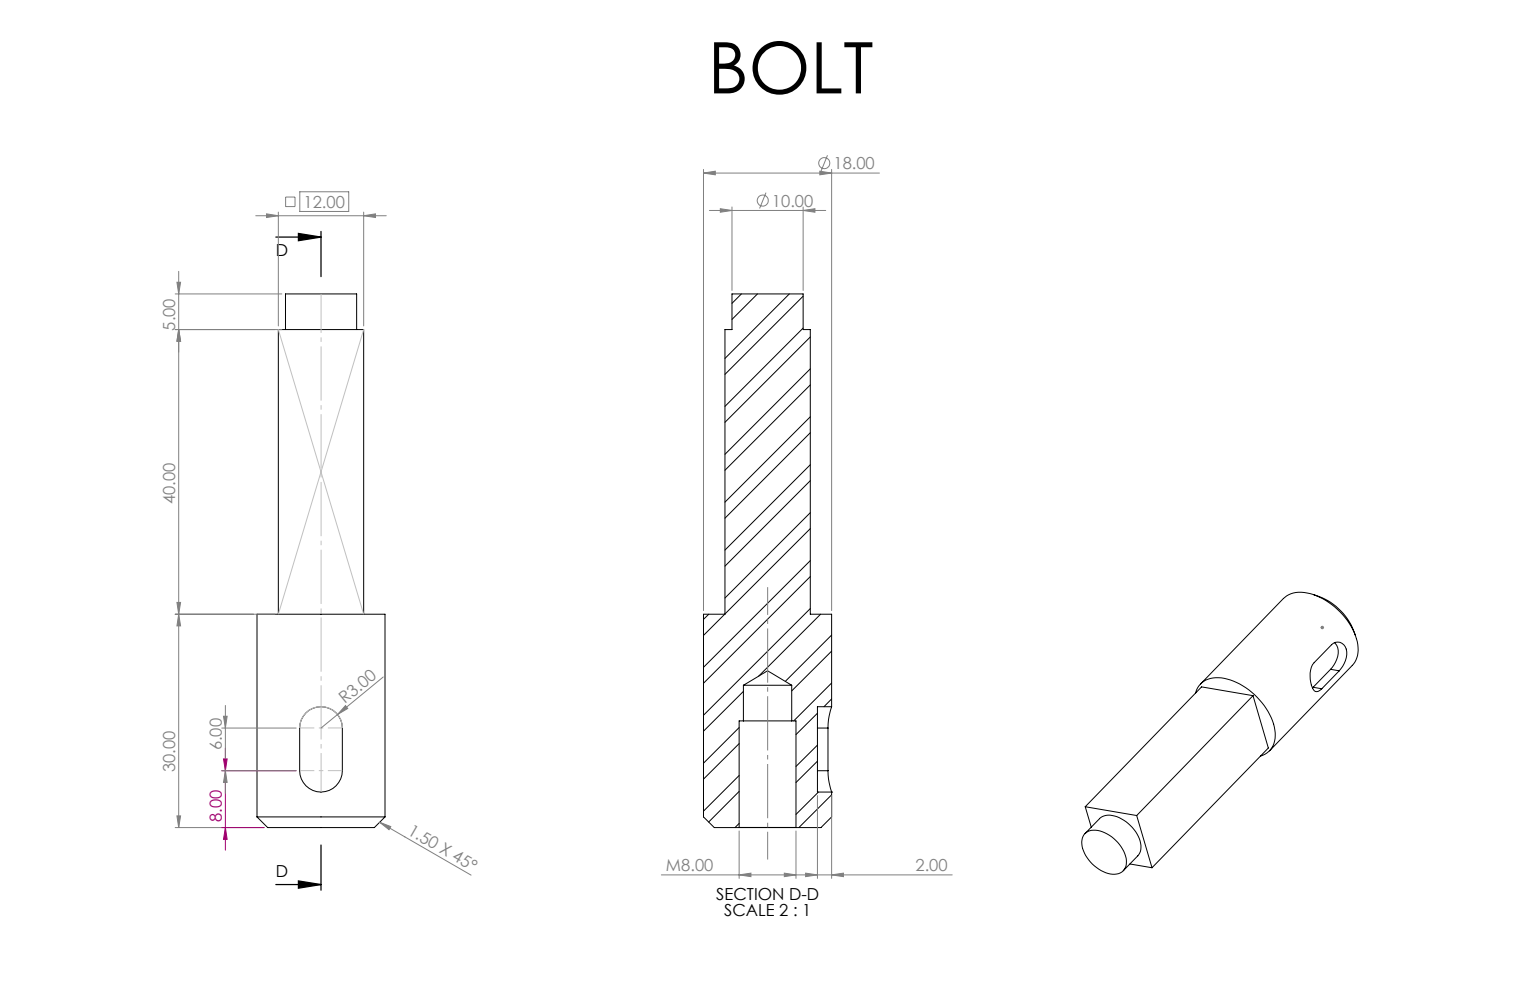
ISO-10303-21;
HEADER;
FILE_DESCRIPTION (('STEP AP214'),
    '1' );
FILE_NAME ('BOLT.step',
    '2026-10-24T00:51:42',
    ( '' ),
    ( '' ),
    'SwSTEP 2.0',
    'SolidWorks 2025',
    '' );
FILE_SCHEMA (( 'AUTOMOTIVE_DESIGN' ));
ENDSEC;

DATA;
#36=CARTESIAN_POINT ( 'NONE',  ( -2.396330562663482766, 23.84645203474120478, 6.679745199209158102 ) ) ;
#83=CIRCLE ( 'NONE', #6686, 8.999999999999998224 ) ;
#86=DIRECTION ( 'NONE',  ( -0.000000000000000000, -1.000000000000000000, -0.000000000000000000 ) ) ;
#93=DIRECTION ( 'NONE',  ( 1.445602896647339163E-16, -0.000000000000000000, 1.000000000000000000 ) ) ;
#98=ORIENTED_EDGE ( 'NONE', *, *, #9067, .T. ) ;
#99=ADVANCED_FACE ( 'NONE', ( #13698 ), #18767, .T. ) ;
#106=CARTESIAN_POINT ( 'NONE',  ( -1.568459684869329074, 24.67391323485165699, 8.880481854261958574 ) ) ;
#156=PLANE ( 'NONE',  #2303 ) ;
#166=FACE_OUTER_BOUND ( 'NONE', #9561, .T. ) ;
#189=EDGE_CURVE ( 'NONE', #17751, #16070, #1466, .T. ) ;
#233=DIRECTION ( 'NONE',  ( 0.000000000000000000, -1.000000000000000000, 0.000000000000000000 ) ) ;
#248=AXIS2_PLACEMENT_3D ( 'NONE', #3692, #16267, #11111 ) ;
#261=CARTESIAN_POINT ( 'NONE',  ( -2.999999999999999112, 30.00000000000000000, 8.485281374238567764 ) ) ;
#308=DIRECTION ( 'NONE',  ( 0.000000000000000000, -1.000000000000000000, 0.000000000000000000 ) ) ;
#314=CARTESIAN_POINT ( 'NONE',  ( -2.999999999999999112, 22.00000000000000355, 8.485281374238567764 ) ) ;
#401=CARTESIAN_POINT ( 'NONE',  ( 5.999999999999999112, -40.00000000000000000, -6.000000000000000000 ) ) ;
#470=ORIENTED_EDGE ( 'NONE', *, *, #21249, .T. ) ;
#514=B_SPLINE_CURVE_WITH_KNOTS ( 'NONE', 3,
 ( #8417, #8302, #13318, #978, #8189, #9907, #4423, #14934, #20459, #1094, #8087, #15044, #13658, #22301, #18383, #11517, #6251, #4767, #6589, #13209, #1429, #17113 ),
 .UNSPECIFIED., .F., .F.,
 ( 4, 2, 2, 2, 2, 2, 2, 2, 2, 2, 4 ),
 ( 0.000000000000000000, 0.1249999999999998612, 0.2499999999999997224, 0.3749999999999995559, 0.4374999999999996114, 0.4999999999999996669, 0.6249999999999996669, 0.7499999999999995559, 0.8749999999999995559, 0.9374999999999998890, 1.000000000000000000 ),
 .UNSPECIFIED. ) ;
#528=VECTOR ( 'NONE', #1528, 1000.000000000000000 ) ;
#533=AXIS2_PLACEMENT_3D ( 'NONE', #17654, #5513, #15925 ) ;
#542=CARTESIAN_POINT ( 'NONE',  ( 1.568459684869332627, 13.32608676514834301, 6.880481854261958574 ) ) ;
#544=DIRECTION ( 'NONE',  ( -0.000000000000000000, 1.000000000000000000, -0.000000000000000000 ) ) ;
#580=VECTOR ( 'NONE', #14375, 1000.000000000000000 ) ;
#666=AXIS2_PLACEMENT_3D ( 'NONE', #5556, #12535, #9120 ) ;
#682=AXIS2_PLACEMENT_3D ( 'NONE', #13089, #4934, #8373 ) ;
#708=ORIENTED_EDGE ( 'NONE', *, *, #21758, .F. ) ;
#722=CARTESIAN_POINT ( 'NONE',  ( -2.673152730111970410, 23.56975547524771741, 8.612623190900162484 ) ) ;
#730=EDGE_CURVE ( 'NONE', #17893, #10226, #5782, .T. ) ;
#783=ORIENTED_EDGE ( 'NONE', *, *, #13913, .T. ) ;
#802=FACE_OUTER_BOUND ( 'NONE', #3383, .T. ) ;
#813=ORIENTED_EDGE ( 'NONE', *, *, #21249, .F. ) ;
#815=EDGE_CURVE ( 'NONE', #15823, #14245, #10221, .T. ) ;
#916=VECTOR ( 'NONE', #20039, 1000.000000000000000 ) ;
#930=EDGE_CURVE ( 'NONE', #7391, #7282, #17354, .T. ) ;
#942=LINE ( 'NONE', #2210, #14631 ) ;
#978=CARTESIAN_POINT ( 'NONE',  ( -2.615521992622583891, 14.48472893833976016, 6.613019222488492943 ) ) ;
#985=CARTESIAN_POINT ( 'NONE',  ( 0.000000000000000000, 9.999999999999998224, 0.000000000000000000 ) ) ;
#1056=CARTESIAN_POINT ( 'NONE',  ( 0.000000000000000000, -40.00000000000000000, 0.000000000000000000 ) ) ;
#1057=CARTESIAN_POINT ( 'NONE',  ( 0.003185071962414435728, 24.99999830921895594, 8.999999436406460163 ) ) ;
#1061=ORIENTED_EDGE ( 'NONE', *, *, #730, .T. ) ;
#1094=CARTESIAN_POINT ( 'NONE',  ( -0.3961047786457937980, 13.02071089460816822, 6.993377406885125325 ) ) ;
#1108=ORIENTED_EDGE ( 'NONE', *, *, #189, .F. ) ;
#1124=DIRECTION ( 'NONE',  ( -0.000000000000000000, 1.000000000000000000, -0.000000000000000000 ) ) ;
#1131=EDGE_LOOP ( 'NONE', ( #16120, #1991 ) ) ;
#1134=ORIENTED_EDGE ( 'NONE', *, *, #7502, .T. ) ;
#1138=EDGE_CURVE ( 'NONE', #16070, #18599, #7758, .T. ) ;
#1211=ORIENTED_EDGE ( 'NONE', *, *, #10301, .T. ) ;
#1231=CARTESIAN_POINT ( 'NONE',  ( 4.929203366568097207E-16, 30.00000000000000355, -4.025000000000000355 ) ) ;
#1292=CARTESIAN_POINT ( 'NONE',  ( 4.898587196589407898E-16, 15.00000000000000355, -3.999999999999994671 ) ) ;
#1324=AXIS2_PLACEMENT_3D ( 'NONE', #6164, #9590, #20145 ) ;
#1347=AXIS2_PLACEMENT_3D ( 'NONE', #14150, #308, #21281 ) ;
#1363=LINE ( 'NONE', #3328, #8712 ) ;
#1385=ORIENTED_EDGE ( 'NONE', *, *, #21758, .T. ) ;
#1393=ORIENTED_EDGE ( 'NONE', *, *, #3282, .F. ) ;
#1429=CARTESIAN_POINT ( 'NONE',  ( 2.999964809120486908, 15.80129619923657103, 6.485293816093339103 ) ) ;
#1466=LINE ( 'NONE', #1231, #11872 ) ;
#1492=VECTOR ( 'NONE', #14249, 1000.000000000000000 ) ;
#1528=DIRECTION ( 'NONE',  ( -1.445602896647339163E-16, -0.000000000000000000, -1.000000000000000000 ) ) ;
#1541=ORIENTED_EDGE ( 'NONE', *, *, #20668, .T. ) ;
#1546=DIRECTION ( 'NONE',  ( 0.000000000000000000, 1.000000000000000000, 0.000000000000000000 ) ) ;
#1556=EDGE_LOOP ( 'NONE', ( #12338, #1541, #14784, #10779 ) ) ;
#1563=VECTOR ( 'NONE', #2236, 1000.000000000000000 ) ;
#1566=B_SPLINE_CURVE_WITH_KNOTS ( 'NONE', 3,
 ( #21891, #18094, #6068, #20054, #2642, #9614 ),
 .UNSPECIFIED., .F., .F.,
 ( 4, 2, 4 ),
 ( 0.5000000000000000000, 0.7500000000000000000, 1.000000000000000000 ),
 .UNSPECIFIED. ) ;
#1580=AXIS2_PLACEMENT_3D ( 'NONE', #3741, #21487, #2586 ) ;
#1593=CONICAL_SURFACE ( 'NONE', #11103, 3.399999999999995026, 1.029744258676652313 ) ;
#1594=EDGE_LOOP ( 'NONE', ( #6227, #6035, #12984, #4629 ) ) ;
#1598=EDGE_CURVE ( 'NONE', #12848, #7247, #8512, .T. ) ;
#1605=CYLINDRICAL_SURFACE ( 'NONE', #682, 3.399999999999995026 ) ;
#1618=EDGE_CURVE ( 'NONE', #18735, #18629, #14479, .T. ) ;
#1648=CARTESIAN_POINT ( 'NONE',  ( 0.000000000000000000, 0.000000000000000000, 0.000000000000000000 ) ) ;
#1653=DIRECTION ( 'NONE',  ( 0.000000000000000000, 1.000000000000000000, 0.000000000000000000 ) ) ;
#1676=ORIENTED_EDGE ( 'NONE', *, *, #17223, .F. ) ;
#1707=EDGE_LOOP ( 'NONE', ( #708, #14419, #2679, #4198, #18260, #21957, #20036, #20335 ) ) ;
#1724=AXIS2_PLACEMENT_3D ( 'NONE', #15557, #93, #5162 ) ;
#1763=( LENGTH_UNIT ( ) NAMED_UNIT ( * ) SI_UNIT ( .MILLI., .METRE. ) );
#1768=CARTESIAN_POINT ( 'NONE',  ( 0.000000000000000000, 30.00000000000000000, 0.000000000000000000 ) ) ;
#1780=ORIENTED_EDGE ( 'NONE', *, *, #6189, .T. ) ;
#1781=CARTESIAN_POINT ( 'NONE',  ( 0.000000000000000000, 30.00000000000000000, 0.000000000000000000 ) ) ;
#1803=EDGE_CURVE ( 'NONE', #13632, #20362, #5094, .T. ) ;
#1843=CARTESIAN_POINT ( 'NONE',  ( 2.999999999999998668, 22.79878727884707956, 6.485281374238567764 ) ) ;
#1865=ORIENTED_EDGE ( 'NONE', *, *, #5944, .F. ) ;
#1891=ADVANCED_FACE ( 'NONE', ( #10334, #3487 ), #6584, .T. ) ;
#1929=FACE_OUTER_BOUND ( 'NONE', #11415, .T. ) ;
#1935=CARTESIAN_POINT ( 'NONE',  ( 0.000000000000000000, -40.00000000000000000, 5.000000000000000000 ) ) ;
#1945=CARTESIAN_POINT ( 'NONE',  ( 2.999999999999998668, 22.79878727884707956, 8.485281374238567764 ) ) ;
#1960=CARTESIAN_POINT ( 'NONE',  ( 0.000000000000000000, 30.00000000000000355, 0.000000000000000000 ) ) ;
#1991=ORIENTED_EDGE ( 'NONE', *, *, #15486, .T. ) ;
#1994=CARTESIAN_POINT ( 'NONE',  ( -2.999999999999998668, 22.00000000000000355, 6.485281374238567764 ) ) ;
#2060=CARTESIAN_POINT ( 'NONE',  ( 0.7921581640248794853, 24.99916066338866116, 6.999720221269573273 ) ) ;
#2073=DIRECTION ( 'NONE',  ( -0.000000000000000000, 1.000000000000000000, -0.000000000000000000 ) ) ;
#2090=ORIENTED_EDGE ( 'NONE', *, *, #14922, .F. ) ;
#2106=AXIS2_PLACEMENT_3D ( 'NONE', #7588, #2317, #7363 ) ;
#2130=DIRECTION ( 'NONE',  ( 0.000000000000000000, 0.000000000000000000, 1.000000000000000000 ) ) ;
#2158=DIRECTION ( 'NONE',  ( -0.000000000000000000, 1.000000000000000000, -0.000000000000000000 ) ) ;
#2171=CARTESIAN_POINT ( 'NONE',  ( 5.999999999999999112, -40.00000000000000000, -6.000000000000000000 ) ) ;
#2210=CARTESIAN_POINT ( 'NONE',  ( -3.000000000000000000, 16.00000000000000000, 8.485281374238567764 ) ) ;
#2236=DIRECTION ( 'NONE',  ( 0.000000000000000000, 0.000000000000000000, -1.000000000000000000 ) ) ;
#2240=ORIENTED_EDGE ( 'NONE', *, *, #12614, .F. ) ;
#2245=PRODUCT_DEFINITION_CONTEXT ( 'detailed design', #5637, 'design' ) ;
#2303=AXIS2_PLACEMENT_3D ( 'NONE', #22413, #10246, #8983 ) ;
#2311=ADVANCED_FACE ( 'NONE', ( #15795 ), #22083, .T. ) ;
#2317=DIRECTION ( 'NONE',  ( 0.000000000000000000, -1.000000000000000000, 0.000000000000000000 ) ) ;
#2331=DIRECTION ( 'NONE',  ( -0.000000000000000000, -1.000000000000000000, -0.000000000000000000 ) ) ;
#2337=ORIENTED_EDGE ( 'NONE', *, *, #18707, .F. ) ;
#2371=EDGE_CURVE ( 'NONE', #4794, #18735, #1566, .T. ) ;
#2417=DIRECTION ( 'NONE',  ( 0.000000000000000000, 0.000000000000000000, 1.000000000000000000 ) ) ;
#2437=ORIENTED_EDGE ( 'NONE', *, *, #11521, .T. ) ;
#2476=DIRECTION ( 'NONE',  ( 0.000000000000000000, 0.7071067811865721087, 0.7071067811865230368 ) ) ;
#2586=DIRECTION ( 'NONE',  ( -1.000000000000000000, 0.000000000000000000, 1.445602896647339163E-16 ) ) ;
#2587=PLANE ( 'NONE',  #8818 ) ;
#2592=ORIENTED_EDGE ( 'NONE', *, *, #16916, .F. ) ;
#2595=CARTESIAN_POINT ( 'NONE',  ( 2.999999999999998668, 22.79878727884707956, 8.485281374238567764 ) ) ;
#2603=ADVANCED_FACE ( 'NONE', ( #17822 ), #21265, .F. ) ;
#2642=CARTESIAN_POINT ( 'NONE',  ( 3.000000000000000444, 15.20112712106396913, 8.485281374238567764 ) ) ;
#2679=ORIENTED_EDGE ( 'NONE', *, *, #3365, .T. ) ;
#2685=ORIENTED_EDGE ( 'NONE', *, *, #6152, .T. ) ;
#2702=CARTESIAN_POINT ( 'NONE',  ( -2.999999999999998668, 22.00000000000000355, 8.485281374238567764 ) ) ;
#2704=CARTESIAN_POINT ( 'NONE',  ( -3.000000000000000000, 16.00000000000000000, 8.485281374238567764 ) ) ;
#2777=DIRECTION ( 'NONE',  ( 0.000000000000000000, -1.000000000000000000, 0.000000000000000000 ) ) ;
#2797=AXIS2_PLACEMENT_3D ( 'NONE', #1781, #5537, #15958 ) ;
#2810=EDGE_LOOP ( 'NONE', ( #18690, #10329 ) ) ;
#2816=CARTESIAN_POINT ( 'NONE',  ( 1.568459684869332627, 13.32608676514834301, 8.880481854261958574 ) ) ;
#2852=EDGE_CURVE ( 'NONE', #11430, #14282, #3269, .T. ) ;
#2860=VECTOR ( 'NONE', #86, 1000.000000000000000 ) ;
#2866=VECTOR ( 'NONE', #10233, 1000.000000000000000 ) ;
#2930=CARTESIAN_POINT ( 'NONE',  ( 2.615521992591937295, 23.51527106174855675, 6.613019222498396132 ) ) ;
#2935=CARTESIAN_POINT ( 'NONE',  ( 3.000000000000000888, 15.99999999999999645, 6.485281374238567764 ) ) ;
#2957=VERTEX_POINT ( 'NONE', #16411 ) ;
#3019=CARTESIAN_POINT ( 'NONE',  ( -6.000000000000000888, 0.000000000000000000, -5.999999999999998224 ) ) ;
#3036=DIRECTION ( 'NONE',  ( 1.000000000000000000, -0.000000000000000000, 0.000000000000000000 ) ) ;
#3045=CARTESIAN_POINT ( 'NONE',  ( -6.000000000000000888, -40.00000000000000000, -5.999999999999998224 ) ) ;
#3073=DIRECTION ( 'NONE',  ( 0.000000000000000000, -0.000000000000000000, -1.000000000000000000 ) ) ;
#3098=VECTOR ( 'NONE', #4298, 1000.000000000000000 ) ;
#3178=DIRECTION ( 'NONE',  ( -0.000000000000000000, 1.000000000000000000, -0.000000000000000000 ) ) ;
#3192=CARTESIAN_POINT ( 'NONE',  ( 0.000000000000000000, -45.00000000000000000, 0.000000000000000000 ) ) ;
#3198=AXIS2_PLACEMENT_3D ( 'NONE', #12267, #10539, #19046 ) ;
#3208=CARTESIAN_POINT ( 'NONE',  ( 0.000000000000000000, 30.00000000000000000, 0.000000000000000000 ) ) ;
#3265=CARTESIAN_POINT ( 'NONE',  ( -1.845281852317813165, 24.39721667535817673, 6.813359845952963845 ) ) ;
#3269=LINE ( 'NONE', #15614, #2866 ) ;
#3282=EDGE_CURVE ( 'NONE', #6865, #17042, #10930, .T. ) ;
#3284=FACE_OUTER_BOUND ( 'NONE', #20720, .T. ) ;
#3328=CARTESIAN_POINT ( 'NONE',  ( 0.000000000000000000, 30.00000000000000000, -7.500000000000000000 ) ) ;
#3347=CYLINDRICAL_SURFACE ( 'NONE', #13196, 8.999999999999998224 ) ;
#3360=DIRECTION ( 'NONE',  ( 1.445602896647339163E-16, 0.000000000000000000, 1.000000000000000000 ) ) ;
#3365=EDGE_CURVE ( 'NONE', #7282, #14700, #4838, .T. ) ;
#3373=ORIENTED_EDGE ( 'NONE', *, *, #9001, .T. ) ;
#3374=CARTESIAN_POINT ( 'NONE',  ( -2.900269772763596876, 22.78549972664023215, 6.519988159899003932 ) ) ;
#3383=EDGE_LOOP ( 'NONE', ( #9239, #2437, #2685, #17262 ) ) ;
#3487=FACE_OUTER_BOUND ( 'NONE', #1131, .T. ) ;
#3592=CIRCLE ( 'NONE', #12346, 5.000000000000000000 ) ;
#3615=VECTOR ( 'NONE', #10576, 1000.000000000000000 ) ;
#3642=EDGE_LOOP ( 'NONE', ( #15490, #98, #17559 ) ) ;
#3683=CARTESIAN_POINT ( 'NONE',  ( -2.673152730111970410, 23.56975547524771741, 6.612623190900161596 ) ) ;
#3692=CARTESIAN_POINT ( 'NONE',  ( 0.000000000000000000, 30.00000000000000000, 0.000000000000000000 ) ) ;
#3699=LINE ( 'NONE', #3045, #10172 ) ;
#3702=ADVANCED_FACE ( 'NONE', ( #802 ), #13255, .F. ) ;
#3705=EDGE_CURVE ( 'NONE', #7282, #7391, #83, .T. ) ;
#3706=ORIENTED_EDGE ( 'NONE', *, *, #4297, .T. ) ;
#3741=CARTESIAN_POINT ( 'NONE',  ( 5.999999999999999112, -40.00000000000000000, -6.000000000000000000 ) ) ;
#3759=EDGE_CURVE ( 'NONE', #3823, #19682, #22455, .T. ) ;
#3761=LINE ( 'NONE', #314, #16607 ) ;
#3821=EDGE_CURVE ( 'NONE', #19682, #15823, #19125, .T. ) ;
#3823=VERTEX_POINT ( 'NONE', #4920 ) ;
#3831=CARTESIAN_POINT ( 'NONE',  ( 0.000000000000000000, 29.97499999999999787, 0.000000000000000000 ) ) ;
#3868=EDGE_CURVE ( 'NONE', #15849, #12848, #19698, .T. ) ;
#3872=CIRCLE ( 'NONE', #17395, 7.500000000000000000 ) ;
#3906=CONICAL_SURFACE ( 'NONE', #1347, 7.500000000000000000, 0.7853981633974447263 ) ;
#4005=PRODUCT_DEFINITION_SHAPE ( 'NONE', 'NONE',  #18657 ) ;
#4023=VERTEX_POINT ( 'NONE', #14625 ) ;
#4028=CARTESIAN_POINT ( 'NONE',  ( -2.673152730111970410, 23.56975547524771741, 8.612623190900162484 ) ) ;
#4081=CARTESIAN_POINT ( 'NONE',  ( 0.000000000000000000, 15.00000000000000000, 0.000000000000000000 ) ) ;
#4177=VECTOR ( 'NONE', #2476, 999.9999999999998863 ) ;
#4198=ORIENTED_EDGE ( 'NONE', *, *, #16916, .T. ) ;
#4285=CARTESIAN_POINT ( 'NONE',  ( 0.000000000000000000, -45.00000000000000000, 5.000000000000000000 ) ) ;
#4297=EDGE_CURVE ( 'NONE', #17042, #6865, #20775, .T. ) ;
#4298=DIRECTION ( 'NONE',  ( 1.049727191138617340E-16, 0.5150380749100560429, -0.8571673007021112234 ) ) ;
#4308=CARTESIAN_POINT ( 'NONE',  ( 4.163799117100996122E-16, 15.00000000000000000, -3.399999999999995914 ) ) ;
#4309=DIRECTION ( 'NONE',  ( 0.000000000000000000, 0.000000000000000000, -1.000000000000000000 ) ) ;
#4399=ORIENTED_EDGE ( 'NONE', *, *, #3759, .T. ) ;
#4423=CARTESIAN_POINT ( 'NONE',  ( -1.516119572518642933, 13.38525031373512064, 6.878942250887981835 ) ) ;
#4425=CARTESIAN_POINT ( 'NONE',  ( 2.673152730111972630, 14.43024452475228614, 6.612623190900158043 ) ) ;
#4434=EDGE_CURVE ( 'NONE', #18399, #11377, #3592, .T. ) ;
#4483=ORIENTED_EDGE ( 'NONE', *, *, #19770, .T. ) ;
#4515=( NAMED_UNIT ( * ) SI_UNIT ( $, .STERADIAN. ) SOLID_ANGLE_UNIT ( ) );
#4538=CARTESIAN_POINT ( 'NONE',  ( -0.7921581640248792633, 13.00083933661134417, 8.999720221269573273 ) ) ;
#4553=EDGE_CURVE ( 'NONE', #17173, #4794, #6860, .T. ) ;
#4586=DIRECTION ( 'NONE',  ( 0.000000000000000000, 0.000000000000000000, 1.000000000000000000 ) ) ;
#4610=ORIENTED_EDGE ( 'NONE', *, *, #7575, .T. ) ;
#4629=ORIENTED_EDGE ( 'NONE', *, *, #930, .F. ) ;
#4647=CARTESIAN_POINT ( 'NONE',  ( 0.000000000000000000, 28.49999999999998934, -8.999999999999998224 ) ) ;
#4724=AXIS2_PLACEMENT_3D ( 'NONE', #6114, #2331, #13076 ) ;
#4731=ORIENTED_EDGE ( 'NONE', *, *, #11521, .F. ) ;
#4748=ORIENTED_EDGE ( 'NONE', *, *, #2371, .T. ) ;
#4767=CARTESIAN_POINT ( 'NONE',  ( 2.842671867368132155, 15.02807304850658987, 6.539645084689668764 ) ) ;
#4793=EDGE_CURVE ( 'NONE', #11430, #19192, #15111, .T. ) ;
#4794=VERTEX_POINT ( 'NONE', #16097 ) ;
#4838=LINE ( 'NONE', #8722, #12759 ) ;
#4872=CARTESIAN_POINT ( 'NONE',  ( -2.670518050928090137, 14.42800760928497539, 8.613211112165400252 ) ) ;
#4889=CARTESIAN_POINT ( 'NONE',  ( -6.000000000000000888, 0.000000000000000000, -5.999999999999998224 ) ) ;
#4907=CARTESIAN_POINT ( 'NONE',  ( 5.999999999999999112, 0.000000000000000000, -6.000000000000000000 ) ) ;
#4920=CARTESIAN_POINT ( 'NONE',  ( -5.999999999999999112, -40.00000000000000000, 6.000000000000001776 ) ) ;
#4934=DIRECTION ( 'NONE',  ( -0.000000000000000000, 1.000000000000000000, -0.000000000000000000 ) ) ;
#4936=EDGE_CURVE ( 'NONE', #20460, #19594, #18693, .T. ) ;
#4942=CARTESIAN_POINT ( 'NONE',  ( -0.003185071962412873176, 13.00000169078104051, 8.999999436406458386 ) ) ;
#4950=VERTEX_POINT ( 'NONE', #2702 ) ;
#4952=CARTESIAN_POINT ( 'NONE',  ( -2.999999999999999112, 16.00000000000000000, 8.485281374238567764 ) ) ;
#4962=EDGE_CURVE ( 'NONE', #4023, #18629, #514, .T. ) ;
#5002=AXIS2_PLACEMENT_3D ( 'NONE', #5712, #9259, #9387 ) ;
#5010=FACE_OUTER_BOUND ( 'NONE', #17802, .T. ) ;
#5046=ORIENTED_EDGE ( 'NONE', *, *, #10998, .T. ) ;
#5067=CARTESIAN_POINT ( 'NONE',  ( -1.572625745558603239, 13.32985487263095159, 8.879522542765043269 ) ) ;
#5094=B_SPLINE_CURVE_WITH_KNOTS ( 'NONE', 3,
 ( #14929, #21954, #6246, #2930, #13202, #9903, #16892, #8185, #15149, #22169, #6469, #13431, #13546, #18840, #3265, #36, #12292, #10564, #3374, #15382, #8410, #5101 ),
 .UNSPECIFIED., .F., .F.,
 ( 4, 2, 2, 2, 2, 2, 2, 2, 2, 2, 4 ),
 ( 0.000000000000000000, 0.1250000000000004163, 0.2500000000000008327, 0.3750000000000012212, 0.4375000000000012212, 0.5000000000000012212, 0.6250000000000012212, 0.7500000000000011102, 0.8750000000000011102, 0.9375000000000005551, 1.000000000000000000 ),
 .UNSPECIFIED. ) ;
#5101=CARTESIAN_POINT ( 'NONE',  ( -2.999999999999998668, 22.00000000000000355, 6.485281374238567764 ) ) ;
#5162=DIRECTION ( 'NONE',  ( 1.000000000000000000, 0.000000000000000000, -1.445602896647339163E-16 ) ) ;
#5349=ORIENTED_EDGE ( 'NONE', *, *, #10128, .T. ) ;
#5451=ORIENTED_EDGE ( 'NONE', *, *, #3821, .F. ) ;
#5461=PLANE ( 'NONE',  #11914 ) ;
#5473=ORIENTED_EDGE ( 'NONE', *, *, #1803, .F. ) ;
#5475=ORIENTED_EDGE ( 'NONE', *, *, #10128, .F. ) ;
#5513=DIRECTION ( 'NONE',  ( -0.000000000000000000, 1.000000000000000000, -0.000000000000000000 ) ) ;
#5537=DIRECTION ( 'NONE',  ( -0.000000000000000000, -1.000000000000000000, -0.000000000000000000 ) ) ;
#5556=CARTESIAN_POINT ( 'NONE',  ( 0.000000000000000000, 30.00000000000000000, 0.000000000000000000 ) ) ;
#5634=ORIENTED_EDGE ( 'NONE', *, *, #3759, .F. ) ;
#5637=APPLICATION_CONTEXT ( 'automotive_design' ) ;
#5694=ORIENTED_EDGE ( 'NONE', *, *, #4553, .T. ) ;
#5696=AXIS2_PLACEMENT_3D ( 'NONE', #9097, #10793, #14580 ) ;
#5708=ORIENTED_EDGE ( 'NONE', *, *, #10301, .F. ) ;
#5712=CARTESIAN_POINT ( 'NONE',  ( 0.000000000000000000, 9.999999999999998224, 0.000000000000000000 ) ) ;
#5728=CARTESIAN_POINT ( 'NONE',  ( 2.999999999999999556, 22.00000000000000000, 6.485281374238567764 ) ) ;
#5767=EDGE_CURVE ( 'NONE', #20460, #7282, #1363, .T. ) ;
#5782=LINE ( 'NONE', #12864, #3098 ) ;
#5821=ADVANCED_FACE ( 'NONE', ( #19126 ), #7241, .T. ) ;
#5854=FACE_OUTER_BOUND ( 'NONE', #10443, .T. ) ;
#5887=FACE_OUTER_BOUND ( 'NONE', #20818, .T. ) ;
#5914=DIRECTION ( 'NONE',  ( -0.000000000000000000, 1.000000000000000000, -0.000000000000000000 ) ) ;
#5937=CARTESIAN_POINT ( 'NONE',  ( 4.929203366568097207E-16, 30.00000000000000355, -4.025000000000000355 ) ) ;
#5944=EDGE_CURVE ( 'NONE', #18599, #16070, #17128, .T. ) ;
#6035=ORIENTED_EDGE ( 'NONE', *, *, #4936, .F. ) ;
#6046=CARTESIAN_POINT ( 'NONE',  ( 5.999999999999999112, -40.00000000000000000, -6.000000000000000000 ) ) ;
#6068=CARTESIAN_POINT ( 'NONE',  ( 1.568459684872858473, 13.32608676515186730, 8.880481854261104147 ) ) ;
#6072=DIRECTION ( 'NONE',  ( 0.000000000000000000, -1.000000000000000000, 0.000000000000000000 ) ) ;
#6094=EDGE_CURVE ( 'NONE', #3823, #18686, #18303, .T. ) ;
#6114=CARTESIAN_POINT ( 'NONE',  ( 0.000000000000000000, 30.00000000000000000, -2.000000000000000000 ) ) ;
#6139=CARTESIAN_POINT ( 'NONE',  ( 2.673152730111972630, 14.43024452475228614, 8.612623190900158932 ) ) ;
#6144=CARTESIAN_POINT ( 'NONE',  ( 0.7921581640149154557, 24.99916066339285692, 8.999720221271109821 ) ) ;
#6152=EDGE_CURVE ( 'NONE', #17751, #14282, #11641, .T. ) ;
#6164=CARTESIAN_POINT ( 'NONE',  ( 0.000000000000000000, 0.000000000000000000, 0.000000000000000000 ) ) ;
#6189=EDGE_CURVE ( 'NONE', #4950, #17173, #13897, .T. ) ;
#6227=ORIENTED_EDGE ( 'NONE', *, *, #10126, .F. ) ;
#6246=CARTESIAN_POINT ( 'NONE',  ( 2.916776610577574314, 22.79308088018310841, 6.515718972866975989 ) ) ;
#6251=CARTESIAN_POINT ( 'NONE',  ( 2.615700731154975145, 14.48345912138648295, 6.612978332551282534 ) ) ;
#6311=ADVANCED_FACE ( 'NONE', ( #5887 ), #21815, .T. ) ;
#6329=DIRECTION ( 'NONE',  ( -0.000000000000000000, 1.000000000000000000, -0.000000000000000000 ) ) ;
#6347=ORIENTED_EDGE ( 'NONE', *, *, #20668, .F. ) ;
#6376=CARTESIAN_POINT ( 'NONE',  ( 6.123233995736766282E-16, -45.00000000000000000, -5.000000000000000000 ) ) ;
#6396=ORIENTED_EDGE ( 'NONE', *, *, #3868, .F. ) ;
#6399=CARTESIAN_POINT ( 'NONE',  ( 0.000000000000000000, 15.00000000000000000, 3.399999999999995470 ) ) ;
#6469=CARTESIAN_POINT ( 'NONE',  ( 0.1993075993174698302, 24.99978691316126955, 6.999930029250658770 ) ) ;
#6502=SHAPE_REPRESENTATION ( 'BOLT', ( #18273 ), #20471 ) ;
#6575=CARTESIAN_POINT ( 'NONE',  ( 6.123233995736766282E-16, -45.00000000000000000, -5.000000000000000000 ) ) ;
#6584=PLANE ( 'NONE',  #7414 ) ;
#6589=CARTESIAN_POINT ( 'NONE',  ( 2.900269772745152519, 15.21450027326556764, 6.519988159905375724 ) ) ;
#6591=CARTESIAN_POINT ( 'NONE',  ( -3.000000000000000000, 16.00000000000000000, 6.485281374238567764 ) ) ;
#6644=EDGE_CURVE ( 'NONE', #4950, #20362, #3761, .T. ) ;
#6685=ORIENTED_EDGE ( 'NONE', *, *, #2371, .F. ) ;
#6686=AXIS2_PLACEMENT_3D ( 'NONE', #21775, #6072, #20059 ) ;
#6703=DIRECTION ( 'NONE',  ( 0.000000000000000000, 1.000000000000000000, 0.000000000000000000 ) ) ;
#6814=ORIENTED_EDGE ( 'NONE', *, *, #7644, .F. ) ;
#6860=B_SPLINE_CURVE_WITH_KNOTS ( 'NONE', 3,
 ( #13515, #18808, #6895, #5067, #10304, #4942 ),
 .UNSPECIFIED., .F., .F.,
 ( 4, 2, 4 ),
 ( 0.000000000000000000, 0.2500000000000000000, 0.5000000000000000000 ),
 .UNSPECIFIED. ) ;
#6865=VERTEX_POINT ( 'NONE', #6376 ) ;
#6874=PLANE ( 'NONE',  #1724 ) ;
#6875=AXIS2_PLACEMENT_3D ( 'NONE', #18101, #14308, #2417 ) ;
#6895=CARTESIAN_POINT ( 'NONE',  ( -2.670518050928090137, 14.42800760928497539, 8.613211112165400252 ) ) ;
#6899=ORIENTED_EDGE ( 'NONE', *, *, #4434, .F. ) ;
#6975=VERTEX_POINT ( 'NONE', #4889 ) ;
#7002=DIRECTION ( 'NONE',  ( -0.000000000000000000, -1.000000000000000000, -0.000000000000000000 ) ) ;
#7035=ORIENTED_EDGE ( 'NONE', *, *, #1803, .T. ) ;
#7067=EDGE_LOOP ( 'NONE', ( #5451, #5634, #17662, #470 ) ) ;
#7082=DIRECTION ( 'NONE',  ( 0.000000000000000000, -1.000000000000000000, 0.000000000000000000 ) ) ;
#7096=LINE ( 'NONE', #7204, #17040 ) ;
#7153=ADVANCED_FACE ( 'NONE', ( #166 ), #12425, .T. ) ;
#7164=ADVANCED_BREP_SHAPE_REPRESENTATION ( '', ( #10851, #18273 ), #20471 ) ;
#7184=EDGE_LOOP ( 'NONE', ( #3706, #17509 ) ) ;
#7188=DIRECTION ( 'NONE',  ( 0.000000000000000000, 0.000000000000000000, -1.000000000000000000 ) ) ;
#7204=CARTESIAN_POINT ( 'NONE',  ( 0.000000000000000000, -45.00000000000000000, 5.000000000000000000 ) ) ;
#7225=ORIENTED_EDGE ( 'NONE', *, *, #1138, .T. ) ;
#7232=VERTEX_POINT ( 'NONE', #401 ) ;
#7241=CONICAL_SURFACE ( 'NONE', #20056, 7.500000000000000000, 0.7853981633974447263 ) ;
#7247=VERTEX_POINT ( 'NONE', #4308 ) ;
#7263=FACE_OUTER_BOUND ( 'NONE', #15492, .T. ) ;
#7282=VERTEX_POINT ( 'NONE', #4647 ) ;
#7286=LINE ( 'NONE', #7624, #1492 ) ;
#7363=DIRECTION ( 'NONE',  ( 0.000000000000000000, 0.000000000000000000, -1.000000000000000000 ) ) ;
#7391=VERTEX_POINT ( 'NONE', #20789 ) ;
#7414=AXIS2_PLACEMENT_3D ( 'NONE', #1768, #20560, #15609 ) ;
#7433=DIRECTION ( 'NONE',  ( 0.000000000000000000, 1.000000000000000000, 0.000000000000000000 ) ) ;
#7451=CARTESIAN_POINT ( 'NONE',  ( -6.000000000000000888, -40.00000000000000000, -5.999999999999998224 ) ) ;
#7502=EDGE_CURVE ( 'NONE', #14282, #17751, #16222, .T. ) ;
#7512=ORIENTED_EDGE ( 'NONE', *, *, #1138, .F. ) ;
#7539=DIRECTION ( 'NONE',  ( 0.000000000000000000, 0.000000000000000000, 1.000000000000000000 ) ) ;
#7567=CYLINDRICAL_SURFACE ( 'NONE', #11988, 5.000000000000000000 ) ;
#7575=EDGE_CURVE ( 'NONE', #14282, #18599, #10942, .T. ) ;
#7579=ADVANCED_FACE ( 'NONE', ( #19439 ), #1593, .F. ) ;
#7588=CARTESIAN_POINT ( 'NONE',  ( 0.000000000000000000, -45.00000000000000000, 0.000000000000000000 ) ) ;
#7595=ORIENTED_EDGE ( 'NONE', *, *, #17800, .F. ) ;
#7624=CARTESIAN_POINT ( 'NONE',  ( 5.999999999999999112, -40.00000000000000000, -6.000000000000000000 ) ) ;
#7644=EDGE_CURVE ( 'NONE', #7232, #17346, #7286, .T. ) ;
#7696=ADVANCED_FACE ( 'NONE', ( #20456 ), #2587, .F. ) ;
#7711=PLANE ( 'NONE',  #19671 ) ;
#7758=CIRCLE ( 'NONE', #16153, 4.025000000000000355 ) ;
#7767=CARTESIAN_POINT ( 'NONE',  ( 4.898587196589408884E-16, 30.00000000000000000, -3.999999999999996447 ) ) ;
#7808=ADVANCED_FACE ( 'NONE', ( #17224, #20904 ), #13774, .F. ) ;
#7835=VECTOR ( 'NONE', #14740, 1000.000000000000000 ) ;
#7846=CARTESIAN_POINT ( 'NONE',  ( 2.999999999999997780, 30.00000000000000000, 8.485281374238567764 ) ) ;
#7851=STYLED_ITEM('',(#22741),#10851);
#7935=DIRECTION ( 'NONE',  ( 0.000000000000000000, 0.000000000000000000, -1.000000000000000000 ) ) ;
#7957=EDGE_CURVE ( 'NONE', #22536, #4950, #18199, .T. ) ;
#8052=EDGE_LOOP ( 'NONE', ( #1676, #17404, #13963, #22249 ) ) ;
#8056=DIRECTION ( 'NONE',  ( 0.000000000000000000, 0.5150380749100560429, 0.8571673007021112234 ) ) ;
#8087=CARTESIAN_POINT ( 'NONE',  ( -0.1993075991723092522, 13.00021308684595311, 6.999930029250709396 ) ) ;
#8094=ADVANCED_FACE ( 'NONE', ( #22482 ), #3347, .T. ) ;
#8116=ORIENTED_EDGE ( 'NONE', *, *, #18280, .F. ) ;
#8118=DIRECTION ( 'NONE',  ( 0.000000000000000000, 0.000000000000000000, 1.000000000000000000 ) ) ;
#8150=ORIENTED_EDGE ( 'NONE', *, *, #15486, .F. ) ;
#8185=CARTESIAN_POINT ( 'NONE',  ( 0.9710767271268372358, 24.84180973946540405, 6.949333411110966807 ) ) ;
#8189=CARTESIAN_POINT ( 'NONE',  ( -2.394928258197305482, 14.15236082731613010, 6.680059847329907541 ) ) ;
#8291=VECTOR ( 'NONE', #9392, 1000.000000000000000 ) ;
#8302=CARTESIAN_POINT ( 'NONE',  ( -2.999929132934958886, 15.60292843345686187, 6.485306429529695826 ) ) ;
#8373=DIRECTION ( 'NONE',  ( 0.000000000000000000, 0.000000000000000000, 1.000000000000000000 ) ) ;
#8410=CARTESIAN_POINT ( 'NONE',  ( -2.999964809119741727, 22.19870380085767891, 6.485293816093604669 ) ) ;
#8417=CARTESIAN_POINT ( 'NONE',  ( -2.999999999999999112, 16.00000000000000000, 6.485281374238567764 ) ) ;
#8453=DIRECTION ( 'NONE',  ( 8.659560562354634570E-17, 0.7071067811865721087, -0.7071067811865230368 ) ) ;
#8478=DIRECTION ( 'NONE',  ( -0.000000000000000000, -1.000000000000000000, -0.000000000000000000 ) ) ;
#8506=CARTESIAN_POINT ( 'NONE',  ( -6.000000000000000888, -40.00000000000000000, -5.999999999999998224 ) ) ;
#8512=CIRCLE ( 'NONE', #17648, 3.399999999999995470 ) ;
#8555=CARTESIAN_POINT ( 'NONE',  ( 4.898587196589410857E-16, 29.97499999999999787, -3.999999999999998224 ) ) ;
#8681=ORIENTED_EDGE ( 'NONE', *, *, #12671, .F. ) ;
#8712=VECTOR ( 'NONE', #17275, 1000.000000000000114 ) ;
#8722=CARTESIAN_POINT ( 'NONE',  ( 0.000000000000000000, 30.00000000000000000, -8.999999999999998224 ) ) ;
#8779=ADVANCED_FACE ( 'NONE', ( #15157 ), #15677, .T. ) ;
#8818=AXIS2_PLACEMENT_3D ( 'NONE', #7846, #3036, #4309 ) ;
#8829=DIRECTION ( 'NONE',  ( 0.000000000000000000, 0.000000000000000000, -1.000000000000000000 ) ) ;
#8906=ADVANCED_FACE ( 'NONE', ( #14453 ), #7711, .T. ) ;
#8912=PLANE ( 'NONE',  #14155 ) ;
#8933=CARTESIAN_POINT ( 'NONE',  ( -0.7857880201000499998, 25.00083595504925071, 9.000278651543347053 ) ) ;
#8940=DIRECTION ( 'NONE',  ( -0.000000000000000000, 1.000000000000000000, -0.000000000000000000 ) ) ;
#8976=CYLINDRICAL_SURFACE ( 'NONE', #2797, 8.999999999999998224 ) ;
#8983=DIRECTION ( 'NONE',  ( 0.000000000000000000, -0.000000000000000000, -1.000000000000000000 ) ) ;
#8990=CONICAL_SURFACE ( 'NONE', #21084, 3.399999999999995026, 1.029744258676652313 ) ;
#9001=EDGE_CURVE ( 'NONE', #20362, #4023, #19863, .T. ) ;
#9003=DIRECTION ( 'NONE',  ( 0.000000000000000000, -1.000000000000000000, 0.000000000000000000 ) ) ;
#9025=CARTESIAN_POINT ( 'NONE',  ( 0.000000000000000000, 9.999999999999998224, 0.000000000000000000 ) ) ;
#9067=EDGE_CURVE ( 'NONE', #17893, #15849, #18253, .T. ) ;
#9093=DIRECTION ( 'NONE',  ( 0.000000000000000000, 0.000000000000000000, -1.000000000000000000 ) ) ;
#9097=CARTESIAN_POINT ( 'NONE',  ( 0.000000000000000000, 30.00000000000000355, 0.000000000000000000 ) ) ;
#9120=DIRECTION ( 'NONE',  ( 0.000000000000000000, 0.000000000000000000, 1.000000000000000000 ) ) ;
#9143=EDGE_CURVE ( 'NONE', #19192, #11430, #10499, .T. ) ;
#9146=DIRECTION ( 'NONE',  ( -1.445602896647339163E-16, 0.000000000000000000, -1.000000000000000000 ) ) ;
#9162=CARTESIAN_POINT ( 'NONE',  ( -2.999999999999999556, 22.00000000000000355, 6.485281374238567764 ) ) ;
#9205=CARTESIAN_POINT ( 'NONE',  ( 0.000000000000000000, 30.00000000000000000, -7.500000000000000000 ) ) ;
#9239=ORIENTED_EDGE ( 'NONE', *, *, #9143, .F. ) ;
#9246=CARTESIAN_POINT ( 'NONE',  ( 3.000000000000000444, 15.20112712106396913, 6.485281374238567764 ) ) ;
#9247=DIRECTION ( 'NONE',  ( 0.000000000000000000, 0.000000000000000000, 1.000000000000000000 ) ) ;
#9259=DIRECTION ( 'NONE',  ( -0.000000000000000000, 1.000000000000000000, -0.000000000000000000 ) ) ;
#9275=ADVANCED_FACE ( 'NONE', ( #19490 ), #10642, .F. ) ;
#9314=AXIS2_PLACEMENT_3D ( 'NONE', #20323, #13187, #20095 ) ;
#9341=ORIENTED_EDGE ( 'NONE', *, *, #12671, .T. ) ;
#9350=ADVANCED_FACE ( 'NONE', ( #12590 ), #7567, .T. ) ;
#9355=DIRECTION ( 'NONE',  ( 0.000000000000000000, 0.000000000000000000, 1.000000000000000000 ) ) ;
#9387=DIRECTION ( 'NONE',  ( 0.000000000000000000, 0.000000000000000000, 1.000000000000000000 ) ) ;
#9388=CARTESIAN_POINT ( 'NONE',  ( 0.000000000000000000, 15.00000000000000355, 3.999999999999994671 ) ) ;
#9392=DIRECTION ( 'NONE',  ( 0.000000000000000000, 1.000000000000000000, 0.000000000000000000 ) ) ;
#9393=EDGE_CURVE ( 'NONE', #11377, #18399, #20416, .T. ) ;
#9394=ORIENTED_EDGE ( 'NONE', *, *, #9067, .F. ) ;
#9402=ORIENTED_EDGE ( 'NONE', *, *, #7644, .T. ) ;
#9418=ADVANCED_FACE ( 'NONE', ( #5854 ), #19731, .T. ) ;
#9561=EDGE_LOOP ( 'NONE', ( #14433, #8681, #9402, #1211 ) ) ;
#9590=DIRECTION ( 'NONE',  ( 0.000000000000000000, 1.000000000000000000, 0.000000000000000000 ) ) ;
#9607=ADVANCED_FACE ( 'NONE', ( #1929 ), #8912, .T. ) ;
#9614=CARTESIAN_POINT ( 'NONE',  ( 2.999999999999997780, 15.99999999999999645, 8.485281374238567764 ) ) ;
#9682=DIRECTION ( 'NONE',  ( 0.000000000000000000, 1.000000000000000000, 0.000000000000000000 ) ) ;
#9728=CIRCLE ( 'NONE', #1324, 8.999999999999998224 ) ;
#9800=CARTESIAN_POINT ( 'NONE',  ( 3.000000000000000444, 15.20112712106396913, 8.485281374238567764 ) ) ;
#9805=CARTESIAN_POINT ( 'NONE',  ( 1.572625745558603905, 24.67014512736903242, 8.879522542765043269 ) ) ;
#9842=CARTESIAN_POINT ( 'NONE',  ( 0.000000000000000000, 29.97499999999999787, 3.999999999999998224 ) ) ;
#9903=CARTESIAN_POINT ( 'NONE',  ( 1.848215538220117304, 24.39449834545646212, 6.812673807617342980 ) ) ;
#9907=CARTESIAN_POINT ( 'NONE',  ( -1.848215538292884208, 13.60550165460329453, 6.812673807599693099 ) ) ;
#9929=LINE ( 'NONE', #7451, #14197 ) ;
#9988=( NAMED_UNIT ( * ) PLANE_ANGLE_UNIT ( ) SI_UNIT ( $, .RADIAN. ) );
#10010=EDGE_LOOP ( 'NONE', ( #4731, #22639, #19473, #1134 ) ) ;
#10022=ORIENTED_EDGE ( 'NONE', *, *, #4962, .F. ) ;
#10126=EDGE_CURVE ( 'NONE', #19594, #7391, #16335, .T. ) ;
#10128=EDGE_CURVE ( 'NONE', #2957, #22536, #11421, .T. ) ;
#10172=VECTOR ( 'NONE', #1546, 1000.000000000000000 ) ;
#10221=LINE ( 'NONE', #17213, #528 ) ;
#10226=VERTEX_POINT ( 'NONE', #20353 ) ;
#10233=DIRECTION ( 'NONE',  ( -0.000000000000000000, 1.000000000000000000, -0.000000000000000000 ) ) ;
#10246=DIRECTION ( 'NONE',  ( 0.000000000000000000, -1.000000000000000000, 0.000000000000000000 ) ) ;
#10251=ORIENTED_EDGE ( 'NONE', *, *, #1618, .F. ) ;
#10297=CARTESIAN_POINT ( 'NONE',  ( 1.010333609296566156E-15, 30.00000000000000000, 7.500000000000000000 ) ) ;
#10301=EDGE_CURVE ( 'NONE', #17346, #6975, #3699, .T. ) ;
#10304=CARTESIAN_POINT ( 'NONE',  ( -0.7921581640149152337, 13.00083933660714663, 8.999720221271109821 ) ) ;
#10329=ORIENTED_EDGE ( 'NONE', *, *, #9143, .T. ) ;
#10334=FACE_BOUND ( 'NONE', #16383, .T. ) ;
#10405=AXIS2_PLACEMENT_3D ( 'NONE', #3192, #15079, #3073 ) ;
#10443=EDGE_LOOP ( 'NONE', ( #10535, #14136, #783, #18117 ) ) ;
#10499=CIRCLE ( 'NONE', #3198, 3.999999999999994671 ) ;
#10516=AXIS2_PLACEMENT_3D ( 'NONE', #15915, #233, #21433 ) ;
#10527=AXIS2_PLACEMENT_3D ( 'NONE', #3831, #14114, #19193 ) ;
#10535=ORIENTED_EDGE ( 'NONE', *, *, #16432, .F. ) ;
#10539=DIRECTION ( 'NONE',  ( -0.000000000000000000, 1.000000000000000000, -0.000000000000000000 ) ) ;
#10548=EDGE_LOOP ( 'NONE', ( #22434, #20899 ) ) ;
#10557=VECTOR ( 'NONE', #12777, 1000.000000000000000 ) ;
#10564=CARTESIAN_POINT ( 'NONE',  ( -2.842671867355789139, 22.97192695149968955, 6.539645084693655797 ) ) ;
#10576=DIRECTION ( 'NONE',  ( -0.000000000000000000, -1.000000000000000000, -0.000000000000000000 ) ) ;
#10586=ORIENTED_EDGE ( 'NONE', *, *, #1618, .T. ) ;
#10588=EDGE_LOOP ( 'NONE', ( #1393, #17001, #15957, #17036 ) ) ;
#10621=LINE ( 'NONE', #12243, #21118 ) ;
#10623=AXIS2_PLACEMENT_3D ( 'NONE', #15275, #9682, #11399 ) ;
#10635=CARTESIAN_POINT ( 'NONE',  ( 1.572625745562107991, 24.67014512736552945, 8.879522542764194171 ) ) ;
#10637=CARTESIAN_POINT ( 'NONE',  ( 0.003185071962414435728, 24.99999830921895594, 8.999999436406460163 ) ) ;
#10642=CYLINDRICAL_SURFACE ( 'NONE', #248, 3.999999999999996447 ) ;
#10694=CARTESIAN_POINT ( 'NONE',  ( 2.999999999999997780, 15.99999999999999645, 8.485281374238567764 ) ) ;
#10779=ORIENTED_EDGE ( 'NONE', *, *, #815, .T. ) ;
#10793=DIRECTION ( 'NONE',  ( -0.000000000000000000, 1.000000000000000000, -0.000000000000000000 ) ) ;
#10830=VECTOR ( 'NONE', #6329, 1000.000000000000000 ) ;
#10849=CARTESIAN_POINT ( 'NONE',  ( 0.000000000000000000, 30.00000000000000000, 3.399999999999995026 ) ) ;
#10851=MANIFOLD_SOLID_BREP ( 'M8 Tapped Hole3', #19569 ) ;
#10870=CARTESIAN_POINT ( 'NONE',  ( -2.999999999999998668, 22.79887287893604153, 8.485281374238567764 ) ) ;
#10908=VECTOR ( 'NONE', #8478, 1000.000000000000000 ) ;
#10930=CIRCLE ( 'NONE', #12036, 5.000000000000000000 ) ;
#10932=ORIENTED_EDGE ( 'NONE', *, *, #15182, .T. ) ;
#10942=LINE ( 'NONE', #21376, #4177 ) ;
#10956=FACE_OUTER_BOUND ( 'NONE', #1594, .T. ) ;
#10968=FACE_OUTER_BOUND ( 'NONE', #11330, .T. ) ;
#10998=EDGE_CURVE ( 'NONE', #7247, #12848, #17358, .T. ) ;
#11048=DIRECTION ( 'NONE',  ( -0.000000000000000000, 1.000000000000000000, -0.000000000000000000 ) ) ;
#11050=CARTESIAN_POINT ( 'NONE',  ( 0.000000000000000000, 9.999999999999998224, 0.000000000000000000 ) ) ;
#11103=AXIS2_PLACEMENT_3D ( 'NONE', #11050, #17821, #2130 ) ;
#11111=DIRECTION ( 'NONE',  ( 0.000000000000000000, 0.000000000000000000, 1.000000000000000000 ) ) ;
#11171=CARTESIAN_POINT ( 'NONE',  ( 2.999999999999998224, 22.00000000000000000, 8.485281374238567764 ) ) ;
#11271=AXIS2_PLACEMENT_3D ( 'NONE', #11648, #3178, #20479 ) ;
#11330=EDGE_LOOP ( 'NONE', ( #9394, #1061, #16025 ) ) ;
#11377=VERTEX_POINT ( 'NONE', #1935 ) ;
#11389=EDGE_LOOP ( 'NONE', ( #5473, #8116, #5349, #11618, #16548 ) ) ;
#11399=DIRECTION ( 'NONE',  ( 0.000000000000000000, 0.000000000000000000, 1.000000000000000000 ) ) ;
#11401=CARTESIAN_POINT ( 'NONE',  ( -1.572625745562107324, 13.32985487263445812, 8.879522542764194171 ) ) ;
#11415=EDGE_LOOP ( 'NONE', ( #15156, #813, #20482, #9341 ) ) ;
#11421=B_SPLINE_CURVE_WITH_KNOTS ( 'NONE', 3,
 ( #11171, #2595, #21725, #9805, #6144, #21967 ),
 .UNSPECIFIED., .F., .F.,
 ( 4, 2, 4 ),
 ( 0.000000000000000000, 0.2500000000000000000, 0.5000000000000000000 ),
 .UNSPECIFIED. ) ;
#11430=VERTEX_POINT ( 'NONE', #9388 ) ;
#11474=AXIS2_PLACEMENT_3D ( 'NONE', #18084, #7433, #19475 ) ;
#11478=CARTESIAN_POINT ( 'NONE',  ( -2.999999999999998668, 22.79887287893604153, 8.485281374238567764 ) ) ;
#11517=CARTESIAN_POINT ( 'NONE',  ( 2.396330562594276348, 14.15354796518962388, 6.679745199225937569 ) ) ;
#11519=CARTESIAN_POINT ( 'NONE',  ( 0.7857880201000516651, 12.99916404495074040, 9.000278651543345276 ) ) ;
#11521=EDGE_CURVE ( 'NONE', #19192, #17751, #14967, .T. ) ;
#11524=CARTESIAN_POINT ( 'NONE',  ( 9.184850993605147944E-16, 30.00000000000000000, 7.500000000000000000 ) ) ;
#11560=ADVANCED_FACE ( 'NONE', ( #13904, #3284 ), #156, .T. ) ;
#11618=ORIENTED_EDGE ( 'NONE', *, *, #7957, .T. ) ;
#11641=CIRCLE ( 'NONE', #10527, 3.999999999999998224 ) ;
#11645=ORIENTED_EDGE ( 'NONE', *, *, #6094, .F. ) ;
#11648=CARTESIAN_POINT ( 'NONE',  ( 0.000000000000000000, 30.00000000000000355, 0.000000000000000000 ) ) ;
#11659=AXIS2_PLACEMENT_3D ( 'NONE', #17850, #544, #7539 ) ;
#11810=DIRECTION ( 'NONE',  ( -0.000000000000000000, -1.000000000000000000, -0.000000000000000000 ) ) ;
#11841=AXIS2_PLACEMENT_3D ( 'NONE', #14819, #14710, #21720 ) ;
#11872=VECTOR ( 'NONE', #8453, 999.9999999999998863 ) ;
#11914=AXIS2_PLACEMENT_3D ( 'NONE', #19785, #9003, #15983 ) ;
#11988=AXIS2_PLACEMENT_3D ( 'NONE', #17884, #8940, #21100 ) ;
#11993=ORIENTED_EDGE ( 'NONE', *, *, #6644, .F. ) ;
#12002=CARTESIAN_POINT ( 'NONE',  ( 2.999999999999997780, 22.00000000000000000, 8.485281374238567764 ) ) ;
#12036=AXIS2_PLACEMENT_3D ( 'NONE', #15699, #15581, #8829 ) ;
#12054=CARTESIAN_POINT ( 'NONE',  ( 0.000000000000000000, 0.000000000000000000, -8.999999999999998224 ) ) ;
#12094=ORIENTED_EDGE ( 'NONE', *, *, #5944, .T. ) ;
#12142=DIRECTION ( 'NONE',  ( -0.000000000000000000, 1.000000000000000000, -0.000000000000000000 ) ) ;
#12169=DIRECTION ( 'NONE',  ( -1.000000000000000000, 0.000000000000000000, 1.445602896647339163E-16 ) ) ;
#12232=CARTESIAN_POINT ( 'NONE',  ( 1.102182119232617517E-15, 30.00000000000000000, 8.999999999999998224 ) ) ;
#12243=CARTESIAN_POINT ( 'NONE',  ( 6.000000000000000888, -40.00000000000000000, 6.000000000000000000 ) ) ;
#12257=CARTESIAN_POINT ( 'NONE',  ( 2.999999999999999556, 22.00000000000000000, 8.485281374238567764 ) ) ;
#12267=CARTESIAN_POINT ( 'NONE',  ( 0.000000000000000000, 15.00000000000000355, 0.000000000000000000 ) ) ;
#12292=CARTESIAN_POINT ( 'NONE',  ( -2.615700731179644301, 23.51654087860100262, 6.612978332543312021 ) ) ;
#12338=ORIENTED_EDGE ( 'NONE', *, *, #16022, .T. ) ;
#12346=AXIS2_PLACEMENT_3D ( 'NONE', #1056, #2777, #19964 ) ;
#12388=ORIENTED_EDGE ( 'NONE', *, *, #10126, .T. ) ;
#12425=PLANE ( 'NONE',  #1580 ) ;
#12535=DIRECTION ( 'NONE',  ( -0.000000000000000000, 1.000000000000000000, -0.000000000000000000 ) ) ;
#12589=CARTESIAN_POINT ( 'NONE',  ( -5.999999999999999112, 0.000000000000000000, 6.000000000000001776 ) ) ;
#12590=FACE_OUTER_BOUND ( 'NONE', #10588, .T. ) ;
#12608=ORIENTED_EDGE ( 'NONE', *, *, #15182, .F. ) ;
#12614=EDGE_CURVE ( 'NONE', #16628, #14700, #22468, .T. ) ;
#12619=CARTESIAN_POINT ( 'NONE',  ( -2.999999999999999112, 30.00000000000000000, 6.485281374238567764 ) ) ;
#12671=EDGE_CURVE ( 'NONE', #7232, #14245, #21415, .T. ) ;
#12759=VECTOR ( 'NONE', #11810, 1000.000000000000000 ) ;
#12777=DIRECTION ( 'NONE',  ( -0.000000000000000000, -1.000000000000000000, -0.000000000000000000 ) ) ;
#12848=VERTEX_POINT ( 'NONE', #6399 ) ;
#12864=CARTESIAN_POINT ( 'NONE',  ( 4.163799117100995136E-16, 9.999999999999998224, -3.399999999999995026 ) ) ;
#12882=VECTOR ( 'NONE', #20607, 1000.000000000000000 ) ;
#12944=PRODUCT ( 'BOLT', 'BOLT', '', ( #19036 ) ) ;
#12984=ORIENTED_EDGE ( 'NONE', *, *, #5767, .T. ) ;
#13001=ORIENTED_EDGE ( 'NONE', *, *, #3365, .F. ) ;
#13013=DIRECTION ( 'NONE',  ( -1.445602896647339163E-16, -0.000000000000000000, -1.000000000000000000 ) ) ;
#13037=DIRECTION ( 'NONE',  ( -0.000000000000000000, 1.000000000000000000, -0.000000000000000000 ) ) ;
#13076=DIRECTION ( 'NONE',  ( 0.000000000000000000, 0.000000000000000000, -1.000000000000000000 ) ) ;
#13089=CARTESIAN_POINT ( 'NONE',  ( 0.000000000000000000, 30.00000000000000000, 0.000000000000000000 ) ) ;
#13107=CARTESIAN_POINT ( 'NONE',  ( 3.000000000000000888, 15.99999999999999645, 8.485281374238567764 ) ) ;
#13111=ADVANCED_FACE ( 'NONE', ( #10956 ), #3906, .T. ) ;
#13187=DIRECTION ( 'NONE',  ( 0.000000000000000000, -1.000000000000000000, 0.000000000000000000 ) ) ;
#13196=AXIS2_PLACEMENT_3D ( 'NONE', #17191, #7002, #17299 ) ;
#13202=CARTESIAN_POINT ( 'NONE',  ( 2.394928258270085930, 23.84763917262409549, 6.680059847312254995 ) ) ;
#13209=CARTESIAN_POINT ( 'NONE',  ( 2.979639132251328260, 15.60364968412344133, 6.492556366676851987 ) ) ;
#13255=CYLINDRICAL_SURFACE ( 'NONE', #17284, 3.999999999999996447 ) ;
#13264=( GEOMETRIC_REPRESENTATION_CONTEXT ( 3 ) GLOBAL_UNCERTAINTY_ASSIGNED_CONTEXT ( ( #19960 ) ) GLOBAL_UNIT_ASSIGNED_CONTEXT ( ( #15026, #9988, #4515 ) ) REPRESENTATION_CONTEXT ( 'NONE', 'WORKASPACE' ) );
#13308=ORIENTED_EDGE ( 'NONE', *, *, #17223, .T. ) ;
#13318=CARTESIAN_POINT ( 'NONE',  ( -2.916776610546922832, 15.20691911972858534, 6.515718972876874737 ) ) ;
#13354=LINE ( 'NONE', #12002, #19746 ) ;
#13431=CARTESIAN_POINT ( 'NONE',  ( -0.3890599827476972639, 25.00042110133432161, 7.000138250718057620 ) ) ;
#13432=ADVANCED_FACE ( 'NONE', ( #7263 ), #18508, .F. ) ;
#13515=CARTESIAN_POINT ( 'NONE',  ( -2.999999999999999112, 16.00000000000000000, 8.485281374238567764 ) ) ;
#13544=( NAMED_UNIT ( * ) PLANE_ANGLE_UNIT ( ) SI_UNIT ( $, .RADIAN. ) );
#13546=CARTESIAN_POINT ( 'NONE',  ( -0.7842774244934771488, 24.91897157216331848, 6.973256348169272201 ) ) ;
#13553=CARTESIAN_POINT ( 'NONE',  ( -3.000000000000000000, 15.20121272115292044, 6.485281374238567764 ) ) ;
#13594=CARTESIAN_POINT ( 'NONE',  ( 6.000000000000000888, 0.000000000000000000, 6.000000000000000000 ) ) ;
#13609=CARTESIAN_POINT ( 'NONE',  ( 1.102182119232617517E-15, 30.00000000000000000, 8.999999999999998224 ) ) ;
#13632=VERTEX_POINT ( 'NONE', #14797 ) ;
#13658=CARTESIAN_POINT ( 'NONE',  ( 0.7842774247521370201, 13.08102842795873677, 6.973256348136009031 ) ) ;
#13695=CARTESIAN_POINT ( 'NONE',  ( 6.123233995736766282E-16, -40.00000000000000000, -5.000000000000000000 ) ) ;
#13698=FACE_OUTER_BOUND ( 'NONE', #7184, .T. ) ;
#13758=FACE_OUTER_BOUND ( 'NONE', #21427, .T. ) ;
#13774=PLANE ( 'NONE',  #15395 ) ;
#13795=ORIENTED_EDGE ( 'NONE', *, *, #15325, .F. ) ;
#13897=LINE ( 'NONE', #15618, #3615 ) ;
#13904=FACE_BOUND ( 'NONE', #22080, .T. ) ;
#13913=EDGE_CURVE ( 'NONE', #17042, #11377, #7096, .T. ) ;
#13963=ORIENTED_EDGE ( 'NONE', *, *, #3868, .T. ) ;
#13982=EDGE_LOOP ( 'NONE', ( #14478, #1385, #5475, #10932, #6685, #19620, #22452, #13001 ) ) ;
#14051=FACE_OUTER_BOUND ( 'NONE', #7067, .T. ) ;
#14114=DIRECTION ( 'NONE',  ( -0.000000000000000000, 1.000000000000000000, -0.000000000000000000 ) ) ;
#14136=ORIENTED_EDGE ( 'NONE', *, *, #4297, .F. ) ;
#14141=LINE ( 'NONE', #16212, #580 ) ;
#14150=CARTESIAN_POINT ( 'NONE',  ( 0.000000000000000000, 30.00000000000000000, 0.000000000000000000 ) ) ;
#14155=AXIS2_PLACEMENT_3D ( 'NONE', #15889, #21183, #9146 ) ;
#14185=CARTESIAN_POINT ( 'NONE',  ( 1.572625745562107991, 24.67014512736552945, 6.879522542764194171 ) ) ;
#14197=VECTOR ( 'NONE', #14423, 1000.000000000000000 ) ;
#14245=VERTEX_POINT ( 'NONE', #4907 ) ;
#14249=DIRECTION ( 'NONE',  ( -1.000000000000000000, 0.000000000000000000, 1.445602896647339163E-16 ) ) ;
#14282=VERTEX_POINT ( 'NONE', #9842 ) ;
#14300=CARTESIAN_POINT ( 'NONE',  ( 2.670518050928090137, 23.57199239071502817, 6.613211112165401140 ) ) ;
#14308=DIRECTION ( 'NONE',  ( -0.000000000000000000, 1.000000000000000000, -0.000000000000000000 ) ) ;
#14375=DIRECTION ( 'NONE',  ( -0.000000000000000000, -1.000000000000000000, -0.000000000000000000 ) ) ;
#14419=ORIENTED_EDGE ( 'NONE', *, *, #930, .T. ) ;
#14423=DIRECTION ( 'NONE',  ( 1.445602896647339163E-16, 0.000000000000000000, 1.000000000000000000 ) ) ;
#14433=ORIENTED_EDGE ( 'NONE', *, *, #16022, .F. ) ;
#14453=FACE_OUTER_BOUND ( 'NONE', #18955, .T. ) ;
#14460=VECTOR ( 'NONE', #20552, 1000.000000000000000 ) ;
#14478=ORIENTED_EDGE ( 'NONE', *, *, #3705, .T. ) ;
#14479=LINE ( 'NONE', #10694, #1563 ) ;
#14580=DIRECTION ( 'NONE',  ( 0.000000000000000000, 0.000000000000000000, 1.000000000000000000 ) ) ;
#14596=ORIENTED_EDGE ( 'NONE', *, *, #189, .T. ) ;
#14598=EDGE_LOOP ( 'NONE', ( #16788, #10251, #12608, #18745 ) ) ;
#14625=CARTESIAN_POINT ( 'NONE',  ( -2.999999999999999112, 16.00000000000000000, 6.485281374238567764 ) ) ;
#14626=DIRECTION ( 'NONE',  ( 1.000000000000000000, -0.000000000000000000, -1.445602896647339163E-16 ) ) ;
#14631=VECTOR ( 'NONE', #7935, 1000.000000000000000 ) ;
#14685=DIRECTION ( 'NONE',  ( 1.000000000000000000, -0.000000000000000000, 0.000000000000000000 ) ) ;
#14700=VERTEX_POINT ( 'NONE', #12054 ) ;
#14710=DIRECTION ( 'NONE',  ( -0.000000000000000000, 1.000000000000000000, -0.000000000000000000 ) ) ;
#14740=DIRECTION ( 'NONE',  ( -0.000000000000000000, 1.000000000000000000, -0.000000000000000000 ) ) ;
#14784=ORIENTED_EDGE ( 'NONE', *, *, #3821, .T. ) ;
#14797=CARTESIAN_POINT ( 'NONE',  ( 2.999999999999998224, 22.00000000000000000, 6.485281374238567764 ) ) ;
#14819=CARTESIAN_POINT ( 'NONE',  ( 0.000000000000000000, 15.00000000000000355, 0.000000000000000000 ) ) ;
#14825=DIRECTION ( 'NONE',  ( 8.659560562354903276E-17, -0.7071067811865500152, 0.7071067811865451302 ) ) ;
#14849=CIRCLE ( 'NONE', #5002, 3.399999999999995026 ) ;
#14922=EDGE_CURVE ( 'NONE', #18686, #7232, #21749, .T. ) ;
#14929=CARTESIAN_POINT ( 'NONE',  ( 2.999999999999998224, 22.00000000000000000, 6.485281374238567764 ) ) ;
#14934=CARTESIAN_POINT ( 'NONE',  ( -0.9710767271268349043, 13.15819026053459240, 6.949333411110965919 ) ) ;
#14967=LINE ( 'NONE', #7767, #7835 ) ;
#14984=CARTESIAN_POINT ( 'NONE',  ( 0.000000000000000000, 30.00000000000000000, 0.000000000000000000 ) ) ;
#15026=( LENGTH_UNIT ( ) NAMED_UNIT ( * ) SI_UNIT ( .MILLI., .METRE. ) );
#15044=CARTESIAN_POINT ( 'NONE',  ( 0.3890599824573822696, 12.99957889865121174, 7.000138250717951927 ) ) ;
#15079=DIRECTION ( 'NONE',  ( 0.000000000000000000, -1.000000000000000000, 0.000000000000000000 ) ) ;
#15111=CIRCLE ( 'NONE', #11841, 3.999999999999994671 ) ;
#15149=CARTESIAN_POINT ( 'NONE',  ( 0.7837852459090882684, 24.89976299354472289, 6.967910395774115528 ) ) ;
#15156=ORIENTED_EDGE ( 'NONE', *, *, #815, .F. ) ;
#15157=FACE_OUTER_BOUND ( 'NONE', #21960, .T. ) ;
#15182=EDGE_CURVE ( 'NONE', #2957, #18735, #14141, .T. ) ;
#15266=( NAMED_UNIT ( * ) SI_UNIT ( $, .STERADIAN. ) SOLID_ANGLE_UNIT ( ) );
#15275=CARTESIAN_POINT ( 'NONE',  ( 0.000000000000000000, 30.00000000000000000, 0.000000000000000000 ) ) ;
#15325=EDGE_CURVE ( 'NONE', #10226, #15849, #15555, .T. ) ;
#15381=ORIENTED_EDGE ( 'NONE', *, *, #6152, .F. ) ;
#15382=CARTESIAN_POINT ( 'NONE',  ( -2.979639132232873688, 22.39635031597078907, 6.492556366683235325 ) ) ;
#15388=EDGE_LOOP ( 'NONE', ( #8150, #12388, #20327, #19968 ) ) ;
#15395=AXIS2_PLACEMENT_3D ( 'NONE', #15724, #1653, #17448 ) ;
#15427=APPLICATION_CONTEXT ( 'automotive_design' ) ;
#15449=FACE_OUTER_BOUND ( 'NONE', #8052, .T. ) ;
#15486=EDGE_CURVE ( 'NONE', #19594, #20460, #3872, .T. ) ;
#15490=ORIENTED_EDGE ( 'NONE', *, *, #730, .F. ) ;
#15491=DIRECTION ( 'NONE',  ( 0.000000000000000000, 0.000000000000000000, 1.000000000000000000 ) ) ;
#15492=EDGE_LOOP ( 'NONE', ( #1108, #19279, #4610, #12094 ) ) ;
#15550=DIRECTION ( 'NONE',  ( 0.000000000000000000, 0.000000000000000000, -1.000000000000000000 ) ) ;
#15555=CIRCLE ( 'NONE', #22179, 3.399999999999995026 ) ;
#15557=CARTESIAN_POINT ( 'NONE',  ( 6.000000000000000888, -40.00000000000000000, 6.000000000000000000 ) ) ;
#15581=DIRECTION ( 'NONE',  ( 0.000000000000000000, -1.000000000000000000, 0.000000000000000000 ) ) ;
#15609=DIRECTION ( 'NONE',  ( 0.000000000000000000, -0.000000000000000000, 1.000000000000000000 ) ) ;
#15614=CARTESIAN_POINT ( 'NONE',  ( 0.000000000000000000, 30.00000000000000000, 3.999999999999996447 ) ) ;
#15618=CARTESIAN_POINT ( 'NONE',  ( -2.999999999999999112, 30.00000000000000000, 8.485281374238567764 ) ) ;
#15624=VECTOR ( 'NONE', #8056, 1000.000000000000000 ) ;
#15677=B_SPLINE_SURFACE_WITH_KNOTS ( 'NONE', 3, 1, ( 
 ( #2704, #6591 ),
 ( #20347, #13553 ),
 ( #4872, #16898 ),
 ( #11401, #18631 ),
 ( #4538, #17002 ),
 ( #11519, #21519 ),
 ( #2816, #542 ),
 ( #6139, #4425 ),
 ( #9800, #9246 ),
 ( #13107, #2935 ) ),
 .UNSPECIFIED., .F., .F., .F.,
 ( 4, 2, 2, 2, 4 ),
 ( 2, 2 ),
 ( 0.000000000000000000, 0.2500000000000000000, 0.5000000000000000000, 0.7500000000000000000, 1.000000000000000000 ),
 ( 0.000000000000000000, 1.000000000000000000 ),
 .UNSPECIFIED. ) ;
#15699=CARTESIAN_POINT ( 'NONE',  ( 0.000000000000000000, -45.00000000000000000, 0.000000000000000000 ) ) ;
#15724=CARTESIAN_POINT ( 'NONE',  ( 0.000000000000000000, 0.000000000000000000, 0.000000000000000000 ) ) ;
#15795=FACE_OUTER_BOUND ( 'NONE', #11389, .T. ) ;
#15823=VERTEX_POINT ( 'NONE', #17177 ) ;
#15849=VERTEX_POINT ( 'NONE', #16017 ) ;
#15889=CARTESIAN_POINT ( 'NONE',  ( 5.999999999999999112, -40.00000000000000000, -6.000000000000000000 ) ) ;
#15906=CARTESIAN_POINT ( 'NONE',  ( -2.999999999999998668, 22.79887287893604153, 6.485281374238567764 ) ) ;
#15915=CARTESIAN_POINT ( 'NONE',  ( 0.000000000000000000, -40.00000000000000000, 0.000000000000000000 ) ) ;
#15925=DIRECTION ( 'NONE',  ( 0.000000000000000000, 0.000000000000000000, 1.000000000000000000 ) ) ;
#15957=ORIENTED_EDGE ( 'NONE', *, *, #4434, .T. ) ;
#15958=DIRECTION ( 'NONE',  ( 0.000000000000000000, 0.000000000000000000, -1.000000000000000000 ) ) ;
#15971=ORIENTED_EDGE ( 'NONE', *, *, #19770, .F. ) ;
#15974=EDGE_CURVE ( 'NONE', #15849, #10226, #14849, .T. ) ;
#15983=DIRECTION ( 'NONE',  ( 0.000000000000000000, -0.000000000000000000, -1.000000000000000000 ) ) ;
#16004=LINE ( 'NONE', #12232, #2860 ) ;
#16017=CARTESIAN_POINT ( 'NONE',  ( 0.000000000000000000, 9.999999999999998224, 3.399999999999995026 ) ) ;
#16022=EDGE_CURVE ( 'NONE', #14245, #6975, #16360, .T. ) ;
#16025=ORIENTED_EDGE ( 'NONE', *, *, #15325, .T. ) ;
#16070=VERTEX_POINT ( 'NONE', #5937 ) ;
#16097=CARTESIAN_POINT ( 'NONE',  ( -0.003185071962412873176, 13.00000169078104051, 8.999999436406458386 ) ) ;
#16120=ORIENTED_EDGE ( 'NONE', *, *, #4936, .T. ) ;
#16153=AXIS2_PLACEMENT_3D ( 'NONE', #1960, #2073, #19608 ) ;
#16212=CARTESIAN_POINT ( 'NONE',  ( 2.999999999999997780, 30.00000000000000000, 8.485281374238567764 ) ) ;
#16222=CIRCLE ( 'NONE', #16590, 3.999999999999998224 ) ;
#16267=DIRECTION ( 'NONE',  ( -0.000000000000000000, 1.000000000000000000, -0.000000000000000000 ) ) ;
#16335=LINE ( 'NONE', #11524, #20445 ) ;
#16337=LINE ( 'NONE', #17943, #10557 ) ;
#16360=LINE ( 'NONE', #19707, #916 ) ;
#16383=EDGE_LOOP ( 'NONE', ( #1865, #7512 ) ) ;
#16397=VECTOR ( 'NONE', #14626, 1000.000000000000000 ) ;
#16411=CARTESIAN_POINT ( 'NONE',  ( 2.999999999999998224, 22.00000000000000000, 8.485281374238567764 ) ) ;
#16432=EDGE_CURVE ( 'NONE', #6865, #18399, #22281, .T. ) ;
#16478=CARTESIAN_POINT ( 'NONE',  ( 0.000000000000000000, 29.97499999999999787, 0.000000000000000000 ) ) ;
#16548=ORIENTED_EDGE ( 'NONE', *, *, #6644, .T. ) ;
#16590=AXIS2_PLACEMENT_3D ( 'NONE', #16478, #1124, #8118 ) ;
#16607=VECTOR ( 'NONE', #7188, 1000.000000000000000 ) ;
#16628=VERTEX_POINT ( 'NONE', #19287 ) ;
#16788=ORIENTED_EDGE ( 'NONE', *, *, #17800, .T. ) ;
#16837=ADVANCED_FACE ( 'NONE', ( #10968 ), #8990, .F. ) ;
#16882=DIRECTION ( 'NONE',  ( 1.445602896647339163E-16, 0.000000000000000000, 1.000000000000000000 ) ) ;
#16892=CARTESIAN_POINT ( 'NONE',  ( 1.516119572518645597, 24.61474968626487581, 6.878942250887983612 ) ) ;
#16898=CARTESIAN_POINT ( 'NONE',  ( -2.670518050928090137, 14.42800760928497539, 6.613211112165401140 ) ) ;
#16905=CARTESIAN_POINT ( 'NONE',  ( -5.393609312304999323E-15, 7.957073895306289835, 0.000000000000000000 ) ) ;
#16916=EDGE_CURVE ( 'NONE', #14700, #16628, #9728, .T. ) ;
#16993=DIRECTION ( 'NONE',  ( 1.000000000000000000, 0.000000000000000000, 0.000000000000000000 ) ) ;
#17001=ORIENTED_EDGE ( 'NONE', *, *, #16432, .T. ) ;
#17002=CARTESIAN_POINT ( 'NONE',  ( -0.7921581640248792633, 13.00083933661134417, 6.999720221269573273 ) ) ;
#17036=ORIENTED_EDGE ( 'NONE', *, *, #13913, .F. ) ;
#17040=VECTOR ( 'NONE', #12142, 1000.000000000000000 ) ;
#17042=VERTEX_POINT ( 'NONE', #4285 ) ;
#17113=CARTESIAN_POINT ( 'NONE',  ( 2.999999999999998668, 15.99999999999999645, 6.485281374238567764 ) ) ;
#17128=CIRCLE ( 'NONE', #11659, 4.025000000000000355 ) ;
#17173=VERTEX_POINT ( 'NONE', #4952 ) ;
#17177=CARTESIAN_POINT ( 'NONE',  ( 6.000000000000000888, 0.000000000000000000, 6.000000000000000000 ) ) ;
#17191=CARTESIAN_POINT ( 'NONE',  ( 0.000000000000000000, 30.00000000000000000, 0.000000000000000000 ) ) ;
#17213=CARTESIAN_POINT ( 'NONE',  ( 5.999999999999999112, 0.000000000000000000, -6.000000000000000000 ) ) ;
#17223=EDGE_CURVE ( 'NONE', #10226, #7247, #22149, .T. ) ;
#17224=FACE_BOUND ( 'NONE', #1556, .T. ) ;
#17230=CARTESIAN_POINT ( 'NONE',  ( 6.000000000000000888, -40.00000000000000000, 6.000000000000000000 ) ) ;
#17262=ORIENTED_EDGE ( 'NONE', *, *, #2852, .F. ) ;
#17274=CARTESIAN_POINT ( 'NONE',  ( -5.999999999999999112, -40.00000000000000000, 6.000000000000001776 ) ) ;
#17275=DIRECTION ( 'NONE',  ( 0.000000000000000000, -0.7071067811865500152, -0.7071067811865451302 ) ) ;
#17284=AXIS2_PLACEMENT_3D ( 'NONE', #14984, #13037, #4586 ) ;
#17299=DIRECTION ( 'NONE',  ( 0.000000000000000000, 0.000000000000000000, -1.000000000000000000 ) ) ;
#17304=MECHANICAL_DESIGN_GEOMETRIC_PRESENTATION_REPRESENTATION('',(#7851),#13264);
#17346=VERTEX_POINT ( 'NONE', #18223 ) ;
#17354=CIRCLE ( 'NONE', #9314, 8.999999999999998224 ) ;
#17358=CIRCLE ( 'NONE', #533, 3.399999999999995470 ) ;
#17395=AXIS2_PLACEMENT_3D ( 'NONE', #22411, #6703, #20683 ) ;
#17404=ORIENTED_EDGE ( 'NONE', *, *, #15974, .F. ) ;
#17443=SHAPE_REPRESENTATION_RELATIONSHIP ( 'NONE' , 'NONE' ,  #6502, #7164 ) ;
#17448=DIRECTION ( 'NONE',  ( 0.000000000000000000, -0.000000000000000000, 1.000000000000000000 ) ) ;
#17459=FACE_OUTER_BOUND ( 'NONE', #1707, .T. ) ;
#17509=ORIENTED_EDGE ( 'NONE', *, *, #3282, .T. ) ;
#17559=ORIENTED_EDGE ( 'NONE', *, *, #15974, .T. ) ;
#17648=AXIS2_PLACEMENT_3D ( 'NONE', #4081, #11048, #21148 ) ;
#17654=CARTESIAN_POINT ( 'NONE',  ( 0.000000000000000000, 15.00000000000000000, 0.000000000000000000 ) ) ;
#17662=ORIENTED_EDGE ( 'NONE', *, *, #6094, .T. ) ;
#17709=FACE_OUTER_BOUND ( 'NONE', #2810, .T. ) ;
#17751=VERTEX_POINT ( 'NONE', #8555 ) ;
#17773=ORIENTED_EDGE ( 'NONE', *, *, #9393, .F. ) ;
#17800=EDGE_CURVE ( 'NONE', #13632, #18629, #16337, .T. ) ;
#17802=EDGE_LOOP ( 'NONE', ( #15381, #14596, #7225, #21207 ) ) ;
#17821=DIRECTION ( 'NONE',  ( -0.000000000000000000, 1.000000000000000000, -0.000000000000000000 ) ) ;
#17822=FACE_OUTER_BOUND ( 'NONE', #21225, .T. ) ;
#17850=CARTESIAN_POINT ( 'NONE',  ( 0.000000000000000000, 30.00000000000000355, 0.000000000000000000 ) ) ;
#17875=CARTESIAN_POINT ( 'NONE',  ( -2.999999999999999556, 22.00000000000000355, 8.485281374238567764 ) ) ;
#17884=CARTESIAN_POINT ( 'NONE',  ( 0.000000000000000000, -45.00000000000000000, 0.000000000000000000 ) ) ;
#17893=VERTEX_POINT ( 'NONE', #16905 ) ;
#17897=PRODUCT_DEFINITION_FORMATION_WITH_SPECIFIED_SOURCE ( 'ANY', '', #12944, .NOT_KNOWN. ) ;
#17943=CARTESIAN_POINT ( 'NONE',  ( 2.999999999999997780, 30.00000000000000000, 6.485281374238567764 ) ) ;
#18084=CARTESIAN_POINT ( 'NONE',  ( 0.000000000000000000, 0.000000000000000000, 0.000000000000000000 ) ) ;
#18094=CARTESIAN_POINT ( 'NONE',  ( 0.7857880201100436723, 12.99916404495491307, 9.000278651541815833 ) ) ;
#18101=CARTESIAN_POINT ( 'NONE',  ( 0.000000000000000000, -45.00000000000000000, 0.000000000000000000 ) ) ;
#18117=ORIENTED_EDGE ( 'NONE', *, *, #9393, .T. ) ;
#18160=VECTOR ( 'NONE', #3360, 1000.000000000000000 ) ;
#18199=B_SPLINE_CURVE_WITH_KNOTS ( 'NONE', 3,
 ( #1057, #20193, #21804, #722, #11478, #21922 ),
 .UNSPECIFIED., .F., .F.,
 ( 4, 2, 4 ),
 ( 0.5000000000000000000, 0.7500000000000000000, 1.000000000000000000 ),
 .UNSPECIFIED. ) ;
#18223=CARTESIAN_POINT ( 'NONE',  ( -6.000000000000000888, -40.00000000000000000, -5.999999999999998224 ) ) ;
#18253=LINE ( 'NONE', #20200, #15624 ) ;
#18260=ORIENTED_EDGE ( 'NONE', *, *, #19614, .F. ) ;
#18273=AXIS2_PLACEMENT_3D ( 'NONE', #1648, #15491, #16993 ) ;
#18280=EDGE_CURVE ( 'NONE', #2957, #13632, #13354, .T. ) ;
#18303=LINE ( 'NONE', #17230, #16397 ) ;
#18368=UNCERTAINTY_MEASURE_WITH_UNIT (LENGTH_MEASURE( 1.000000000000000082E-05 ), #1763, 'distance_accuracy_value', 'NONE');
#18383=CARTESIAN_POINT ( 'NONE',  ( 1.845281852387030908, 13.60278332471100704, 6.813359845936179049 ) ) ;
#18391=VECTOR ( 'NONE', #22230, 1000.000000000000000 ) ;
#18399=VERTEX_POINT ( 'NONE', #13695 ) ;
#18508=CONICAL_SURFACE ( 'NONE', #5696, 4.025000000000000355, 0.7853981633974136400 ) ;
#18599=VERTEX_POINT ( 'NONE', #19514 ) ;
#18604=LINE ( 'NONE', #3019, #18160 ) ;
#18629=VERTEX_POINT ( 'NONE', #19966 ) ;
#18631=CARTESIAN_POINT ( 'NONE',  ( -1.572625745562107324, 13.32985487263445812, 6.879522542764194171 ) ) ;
#18657=PRODUCT_DEFINITION ( 'UNKNOWN', '', #17897, #2245 ) ;
#18686=VERTEX_POINT ( 'NONE', #21686 ) ;
#18690=ORIENTED_EDGE ( 'NONE', *, *, #4793, .T. ) ;
#18693=CIRCLE ( 'NONE', #10623, 7.500000000000000000 ) ;
#18707=EDGE_CURVE ( 'NONE', #17173, #4023, #942, .T. ) ;
#18735=VERTEX_POINT ( 'NONE', #21457 ) ;
#18745=ORIENTED_EDGE ( 'NONE', *, *, #18280, .T. ) ;
#18767=PLANE ( 'NONE',  #10405 ) ;
#18796=LINE ( 'NONE', #13609, #10908 ) ;
#18808=CARTESIAN_POINT ( 'NONE',  ( -3.000000000000000000, 15.20121272115292044, 8.485281374238567764 ) ) ;
#18840=CARTESIAN_POINT ( 'NONE',  ( -1.511556752833622896, 24.61754848632951465, 6.879730668860025489 ) ) ;
#18925=VECTOR ( 'NONE', #19636, 1000.000000000000000 ) ;
#18955=EDGE_LOOP ( 'NONE', ( #22420, #11993, #1780, #20497 ) ) ;
#19036=PRODUCT_CONTEXT ( 'NONE', #15427, 'mechanical' ) ;
#19046=DIRECTION ( 'NONE',  ( 0.000000000000000000, 0.000000000000000000, 1.000000000000000000 ) ) ;
#19124=ADVANCED_FACE ( 'NONE', ( #13758 ), #20443, .T. ) ;
#19125=LINE ( 'NONE', #13594, #12882 ) ;
#19126=FACE_OUTER_BOUND ( 'NONE', #15388, .T. ) ;
#19192=VERTEX_POINT ( 'NONE', #1292 ) ;
#19193=DIRECTION ( 'NONE',  ( 0.000000000000000000, 0.000000000000000000, 1.000000000000000000 ) ) ;
#19248=DIRECTION ( 'NONE',  ( 0.000000000000000000, 1.000000000000000000, 0.000000000000000000 ) ) ;
#19263=CARTESIAN_POINT ( 'NONE',  ( -0.7857880201000499998, 25.00083595504925071, 7.000278651543347053 ) ) ;
#19279=ORIENTED_EDGE ( 'NONE', *, *, #7502, .F. ) ;
#19287=CARTESIAN_POINT ( 'NONE',  ( 1.102182119232617517E-15, 0.000000000000000000, 8.999999999999998224 ) ) ;
#19439=FACE_OUTER_BOUND ( 'NONE', #3642, .T. ) ;
#19456=ORIENTED_EDGE ( 'NONE', *, *, #4962, .T. ) ;
#19473=ORIENTED_EDGE ( 'NONE', *, *, #2852, .T. ) ;
#19475=DIRECTION ( 'NONE',  ( 0.000000000000000000, 0.000000000000000000, 1.000000000000000000 ) ) ;
#19490=FACE_OUTER_BOUND ( 'NONE', #10010, .T. ) ;
#19514=CARTESIAN_POINT ( 'NONE',  ( 0.000000000000000000, 30.00000000000000355, 4.025000000000000355 ) ) ;
#19560=ADVANCED_FACE ( 'NONE', ( #15449 ), #1605, .F. ) ;
#19569=CLOSED_SHELL ( 'NONE', ( #21952, #3702, #2603, #16837, #9350, #5821, #8094, #20363, #1891, #7808, #13111, #19124, #7153, #9607, #21196, #11560, #9418, #99, #7696, #8779, #8906, #2311, #6311, #7579, #19560, #20049, #9275, #13432 ) ) ;
#19594=VERTEX_POINT ( 'NONE', #10297 ) ;
#19595=CARTESIAN_POINT ( 'NONE',  ( 0.7921581640248794853, 24.99916066338866116, 8.999720221269573273 ) ) ;
#19608=DIRECTION ( 'NONE',  ( 0.000000000000000000, 0.000000000000000000, 1.000000000000000000 ) ) ;
#19614=EDGE_CURVE ( 'NONE', #4794, #16628, #18796, .T. ) ;
#19620=ORIENTED_EDGE ( 'NONE', *, *, #19614, .T. ) ;
#19636=DIRECTION ( 'NONE',  ( -0.000000000000000000, -1.000000000000000000, -0.000000000000000000 ) ) ;
#19671=AXIS2_PLACEMENT_3D ( 'NONE', #261, #14685, #9093 ) ;
#19679=AXIS2_PLACEMENT_3D ( 'NONE', #8506, #12169, #16882 ) ;
#19682=VERTEX_POINT ( 'NONE', #12589 ) ;
#19698=LINE ( 'NONE', #10849, #22426 ) ;
#19707=CARTESIAN_POINT ( 'NONE',  ( 5.999999999999999112, 0.000000000000000000, -6.000000000000000000 ) ) ;
#19723=CARTESIAN_POINT ( 'NONE',  ( 2.670518050928090137, 23.57199239071502817, 8.613211112165400252 ) ) ;
#19731=CYLINDRICAL_SURFACE ( 'NONE', #6875, 5.000000000000000000 ) ;
#19746=VECTOR ( 'NONE', #20488, 1000.000000000000000 ) ;
#19770=EDGE_CURVE ( 'NONE', #17346, #3823, #9929, .T. ) ;
#19785=CARTESIAN_POINT ( 'NONE',  ( 3.399999999999995470, 15.00000000000000178, 0.000000000000000000 ) ) ;
#19863=LINE ( 'NONE', #12619, #18925 ) ;
#19960=UNCERTAINTY_MEASURE_WITH_UNIT (LENGTH_MEASURE( 1.000000000000000082E-05 ), #15026, 'distance_accuracy_value', 'NONE');
#19964=DIRECTION ( 'NONE',  ( 0.000000000000000000, 0.000000000000000000, -1.000000000000000000 ) ) ;
#19966=CARTESIAN_POINT ( 'NONE',  ( 2.999999999999998668, 15.99999999999999645, 6.485281374238567764 ) ) ;
#19968=ORIENTED_EDGE ( 'NONE', *, *, #5767, .F. ) ;
#20036=ORIENTED_EDGE ( 'NONE', *, *, #6189, .F. ) ;
#20039=DIRECTION ( 'NONE',  ( -1.000000000000000000, 0.000000000000000000, 1.445602896647339163E-16 ) ) ;
#20049=ADVANCED_FACE ( 'NONE', ( #21495, #17709 ), #5461, .F. ) ;
#20054=CARTESIAN_POINT ( 'NONE',  ( 2.673152730111972630, 14.43024452475228614, 8.612623190900158932 ) ) ;
#20056=AXIS2_PLACEMENT_3D ( 'NONE', #3208, #7082, #15550 ) ;
#20059=DIRECTION ( 'NONE',  ( 0.000000000000000000, 0.000000000000000000, 1.000000000000000000 ) ) ;
#20095=DIRECTION ( 'NONE',  ( 0.000000000000000000, 0.000000000000000000, 1.000000000000000000 ) ) ;
#20110=EDGE_LOOP ( 'NONE', ( #2592, #2240 ) ) ;
#20145=DIRECTION ( 'NONE',  ( 0.000000000000000000, 0.000000000000000000, 1.000000000000000000 ) ) ;
#20193=CARTESIAN_POINT ( 'NONE',  ( -0.7857880201100420070, 25.00083595504507983, 9.000278651541817609 ) ) ;
#20200=CARTESIAN_POINT ( 'NONE',  ( 0.000000000000000000, 9.999999999999998224, 3.399999999999995026 ) ) ;
#20323=CARTESIAN_POINT ( 'NONE',  ( 0.000000000000000000, 28.49999999999998934, 0.000000000000000000 ) ) ;
#20327=ORIENTED_EDGE ( 'NONE', *, *, #3705, .F. ) ;
#20335=ORIENTED_EDGE ( 'NONE', *, *, #7957, .F. ) ;
#20347=CARTESIAN_POINT ( 'NONE',  ( -3.000000000000000000, 15.20121272115292044, 8.485281374238567764 ) ) ;
#20353=CARTESIAN_POINT ( 'NONE',  ( 4.163799117100995136E-16, 9.999999999999998224, -3.399999999999995026 ) ) ;
#20356=VECTOR ( 'NONE', #13013, 1000.000000000000000 ) ;
#20362=VERTEX_POINT ( 'NONE', #1994 ) ;
#20363=ADVANCED_FACE ( 'NONE', ( #17459 ), #8976, .T. ) ;
#20416=CIRCLE ( 'NONE', #10516, 5.000000000000000000 ) ;
#20443=PLANE ( 'NONE',  #19679 ) ;
#20445=VECTOR ( 'NONE', #14825, 1000.000000000000114 ) ;
#20456=FACE_OUTER_BOUND ( 'NONE', #14598, .T. ) ;
#20459=CARTESIAN_POINT ( 'NONE',  ( -0.7837852459083360923, 13.10023700646259037, 6.967910395774163490 ) ) ;
#20460=VERTEX_POINT ( 'NONE', #9205 ) ;
#20471=( GEOMETRIC_REPRESENTATION_CONTEXT ( 3 ) GLOBAL_UNCERTAINTY_ASSIGNED_CONTEXT ( ( #18368 ) ) GLOBAL_UNIT_ASSIGNED_CONTEXT ( ( #1763, #13544, #15266 ) ) REPRESENTATION_CONTEXT ( 'NONE', 'WORKASPACE' ) );
#20479=DIRECTION ( 'NONE',  ( 0.000000000000000000, 0.000000000000000000, 1.000000000000000000 ) ) ;
#20482=ORIENTED_EDGE ( 'NONE', *, *, #14922, .T. ) ;
#20488=DIRECTION ( 'NONE',  ( 0.000000000000000000, 0.000000000000000000, -1.000000000000000000 ) ) ;
#20497=ORIENTED_EDGE ( 'NONE', *, *, #18707, .T. ) ;
#20552=DIRECTION ( 'NONE',  ( -0.000000000000000000, 1.000000000000000000, -0.000000000000000000 ) ) ;
#20560=DIRECTION ( 'NONE',  ( 0.000000000000000000, 1.000000000000000000, 0.000000000000000000 ) ) ;
#20607=DIRECTION ( 'NONE',  ( 1.000000000000000000, -0.000000000000000000, -1.445602896647339163E-16 ) ) ;
#20668=EDGE_CURVE ( 'NONE', #6975, #19682, #18604, .T. ) ;
#20683=DIRECTION ( 'NONE',  ( 0.000000000000000000, 0.000000000000000000, 1.000000000000000000 ) ) ;
#20720=EDGE_LOOP ( 'NONE', ( #15971, #6814, #2090, #11645 ) ) ;
#20775=CIRCLE ( 'NONE', #2106, 5.000000000000000000 ) ;
#20789=CARTESIAN_POINT ( 'NONE',  ( 1.102182119232617517E-15, 28.49999999999998934, 8.999999999999998224 ) ) ;
#20818=EDGE_LOOP ( 'NONE', ( #7595, #7035, #3373, #19456 ) ) ;
#20899=ORIENTED_EDGE ( 'NONE', *, *, #10998, .F. ) ;
#20904=FACE_OUTER_BOUND ( 'NONE', #20110, .T. ) ;
#21084=AXIS2_PLACEMENT_3D ( 'NONE', #9025, #2158, #9247 ) ;
#21100=DIRECTION ( 'NONE',  ( 0.000000000000000000, 0.000000000000000000, 1.000000000000000000 ) ) ;
#21118=VECTOR ( 'NONE', #19248, 1000.000000000000000 ) ;
#21148=DIRECTION ( 'NONE',  ( 0.000000000000000000, 0.000000000000000000, 1.000000000000000000 ) ) ;
#21183=DIRECTION ( 'NONE',  ( 1.000000000000000000, 0.000000000000000000, -1.445602896647339163E-16 ) ) ;
#21196=ADVANCED_FACE ( 'NONE', ( #14051 ), #6874, .T. ) ;
#21207=ORIENTED_EDGE ( 'NONE', *, *, #7575, .F. ) ;
#21225=EDGE_LOOP ( 'NONE', ( #13795, #13308, #5046, #6396 ) ) ;
#21249=EDGE_CURVE ( 'NONE', #18686, #15823, #10621, .T. ) ;
#21265=CYLINDRICAL_SURFACE ( 'NONE', #666, 3.399999999999995026 ) ;
#21281=DIRECTION ( 'NONE',  ( 0.000000000000000000, 0.000000000000000000, -1.000000000000000000 ) ) ;
#21376=CARTESIAN_POINT ( 'NONE',  ( 0.000000000000000000, 30.00000000000000355, 4.025000000000000355 ) ) ;
#21403=DIRECTION ( 'NONE',  ( -0.000000000000000000, 1.000000000000000000, -0.000000000000000000 ) ) ;
#21415=LINE ( 'NONE', #2171, #8291 ) ;
#21423=CARTESIAN_POINT ( 'NONE',  ( -1.568459684869329074, 24.67391323485165699, 6.880481854261958574 ) ) ;
#21427=EDGE_LOOP ( 'NONE', ( #6347, #5708, #4483, #4399 ) ) ;
#21433=DIRECTION ( 'NONE',  ( 0.000000000000000000, 0.000000000000000000, -1.000000000000000000 ) ) ;
#21457=CARTESIAN_POINT ( 'NONE',  ( 2.999999999999997780, 15.99999999999999645, 8.485281374238567764 ) ) ;
#21487=DIRECTION ( 'NONE',  ( -1.445602896647339163E-16, 0.000000000000000000, -1.000000000000000000 ) ) ;
#21495=FACE_BOUND ( 'NONE', #10548, .T. ) ;
#21519=CARTESIAN_POINT ( 'NONE',  ( 0.7857880201000516651, 12.99916404495074040, 7.000278651543345276 ) ) ;
#21532=CONICAL_SURFACE ( 'NONE', #11271, 4.025000000000000355, 0.7853981633974136400 ) ;
#21686=CARTESIAN_POINT ( 'NONE',  ( 6.000000000000000888, -40.00000000000000000, 6.000000000000000000 ) ) ;
#21720=DIRECTION ( 'NONE',  ( 0.000000000000000000, 0.000000000000000000, 1.000000000000000000 ) ) ;
#21725=CARTESIAN_POINT ( 'NONE',  ( 2.670518050928090137, 23.57199239071502817, 8.613211112165400252 ) ) ;
#21749=LINE ( 'NONE', #6046, #20356 ) ;
#21758=EDGE_CURVE ( 'NONE', #7391, #22536, #16004, .T. ) ;
#21775=CARTESIAN_POINT ( 'NONE',  ( 0.000000000000000000, 28.49999999999998934, 0.000000000000000000 ) ) ;
#21804=CARTESIAN_POINT ( 'NONE',  ( -1.568459684872854920, 24.67391323484813626, 8.880481854261104147 ) ) ;
#21815=CYLINDRICAL_SURFACE ( 'NONE', #4724, 8.999999999999998224 ) ;
#21891=CARTESIAN_POINT ( 'NONE',  ( -0.003185071962412873176, 13.00000169078104051, 8.999999436406458386 ) ) ;
#21922=CARTESIAN_POINT ( 'NONE',  ( -2.999999999999998668, 22.00000000000000355, 8.485281374238567764 ) ) ;
#21952=ADVANCED_FACE ( 'NONE', ( #5010 ), #21532, .F. ) ;
#21954=CARTESIAN_POINT ( 'NONE',  ( 2.999929132934961995, 22.39707156654313991, 6.485306429529692274 ) ) ;
#21957=ORIENTED_EDGE ( 'NONE', *, *, #4553, .F. ) ;
#21960=EDGE_LOOP ( 'NONE', ( #10022, #2337, #5694, #4748, #10586 ) ) ;
#21967=CARTESIAN_POINT ( 'NONE',  ( 0.003185071962414435728, 24.99999830921895594, 8.999999436406460163 ) ) ;
#22080=EDGE_LOOP ( 'NONE', ( #17773, #6899 ) ) ;
#22083=B_SPLINE_SURFACE_WITH_KNOTS ( 'NONE', 3, 1, ( 
 ( #12257, #5728 ),
 ( #1945, #1843 ),
 ( #19723, #14300 ),
 ( #10635, #14185 ),
 ( #19595, #2060 ),
 ( #8933, #19263 ),
 ( #106, #21423 ),
 ( #4028, #3683 ),
 ( #10870, #15906 ),
 ( #17875, #9162 ) ),
 .UNSPECIFIED., .F., .F., .F.,
 ( 4, 2, 2, 2, 4 ),
 ( 2, 2 ),
 ( 0.000000000000000000, 0.2500000000000000000, 0.5000000000000000000, 0.7500000000000000000, 1.000000000000000000 ),
 ( 0.000000000000000000, 1.000000000000000000 ),
 .UNSPECIFIED. ) ;
#22135=SHAPE_DEFINITION_REPRESENTATION ( #4005, #6502 ) ;
#22149=LINE ( 'NONE', #22266, #10830 ) ;
#22169=CARTESIAN_POINT ( 'NONE',  ( 0.3961047786450465069, 24.97928910538451319, 6.993377406885177727 ) ) ;
#22179=AXIS2_PLACEMENT_3D ( 'NONE', #985, #5914, #9355 ) ;
#22230=DIRECTION ( 'NONE',  ( 0.000000000000000000, 1.000000000000000000, 0.000000000000000000 ) ) ;
#22249=ORIENTED_EDGE ( 'NONE', *, *, #1598, .T. ) ;
#22266=CARTESIAN_POINT ( 'NONE',  ( 4.163799117100995136E-16, 30.00000000000000000, -3.399999999999995026 ) ) ;
#22281=LINE ( 'NONE', #6575, #14460 ) ;
#22301=CARTESIAN_POINT ( 'NONE',  ( 1.511556752574976237, 13.38245151354841056, 6.879730668893286882 ) ) ;
#22411=CARTESIAN_POINT ( 'NONE',  ( 0.000000000000000000, 30.00000000000000000, 0.000000000000000000 ) ) ;
#22413=CARTESIAN_POINT ( 'NONE',  ( 0.000000000000000000, -40.00000000000000000, 0.000000000000000000 ) ) ;
#22420=ORIENTED_EDGE ( 'NONE', *, *, #9001, .F. ) ;
#22426=VECTOR ( 'NONE', #21403, 1000.000000000000000 ) ;
#22434=ORIENTED_EDGE ( 'NONE', *, *, #1598, .F. ) ;
#22452=ORIENTED_EDGE ( 'NONE', *, *, #12614, .T. ) ;
#22455=LINE ( 'NONE', #17274, #18391 ) ;
#22468=CIRCLE ( 'NONE', #11474, 8.999999999999998224 ) ;
#22482=FACE_OUTER_BOUND ( 'NONE', #13982, .T. ) ;
#22536=VERTEX_POINT ( 'NONE', #10637 ) ;
#22639=ORIENTED_EDGE ( 'NONE', *, *, #4793, .F. ) ;
#22735=COLOUR_RGB('Black',0.12,0.14,0.17);
#22736=FILL_AREA_STYLE_COLOUR('',#22735);
#22737=FILL_AREA_STYLE('',(#22736));
#22738=SURFACE_STYLE_FILL_AREA(#22737);
#22739=SURFACE_SIDE_STYLE('',(#22738));
#22740=SURFACE_STYLE_USAGE(.BOTH.,#22739);
#22741=PRESENTATION_STYLE_ASSIGNMENT((#22740));
ENDSEC;
END-ISO-10303-21;
